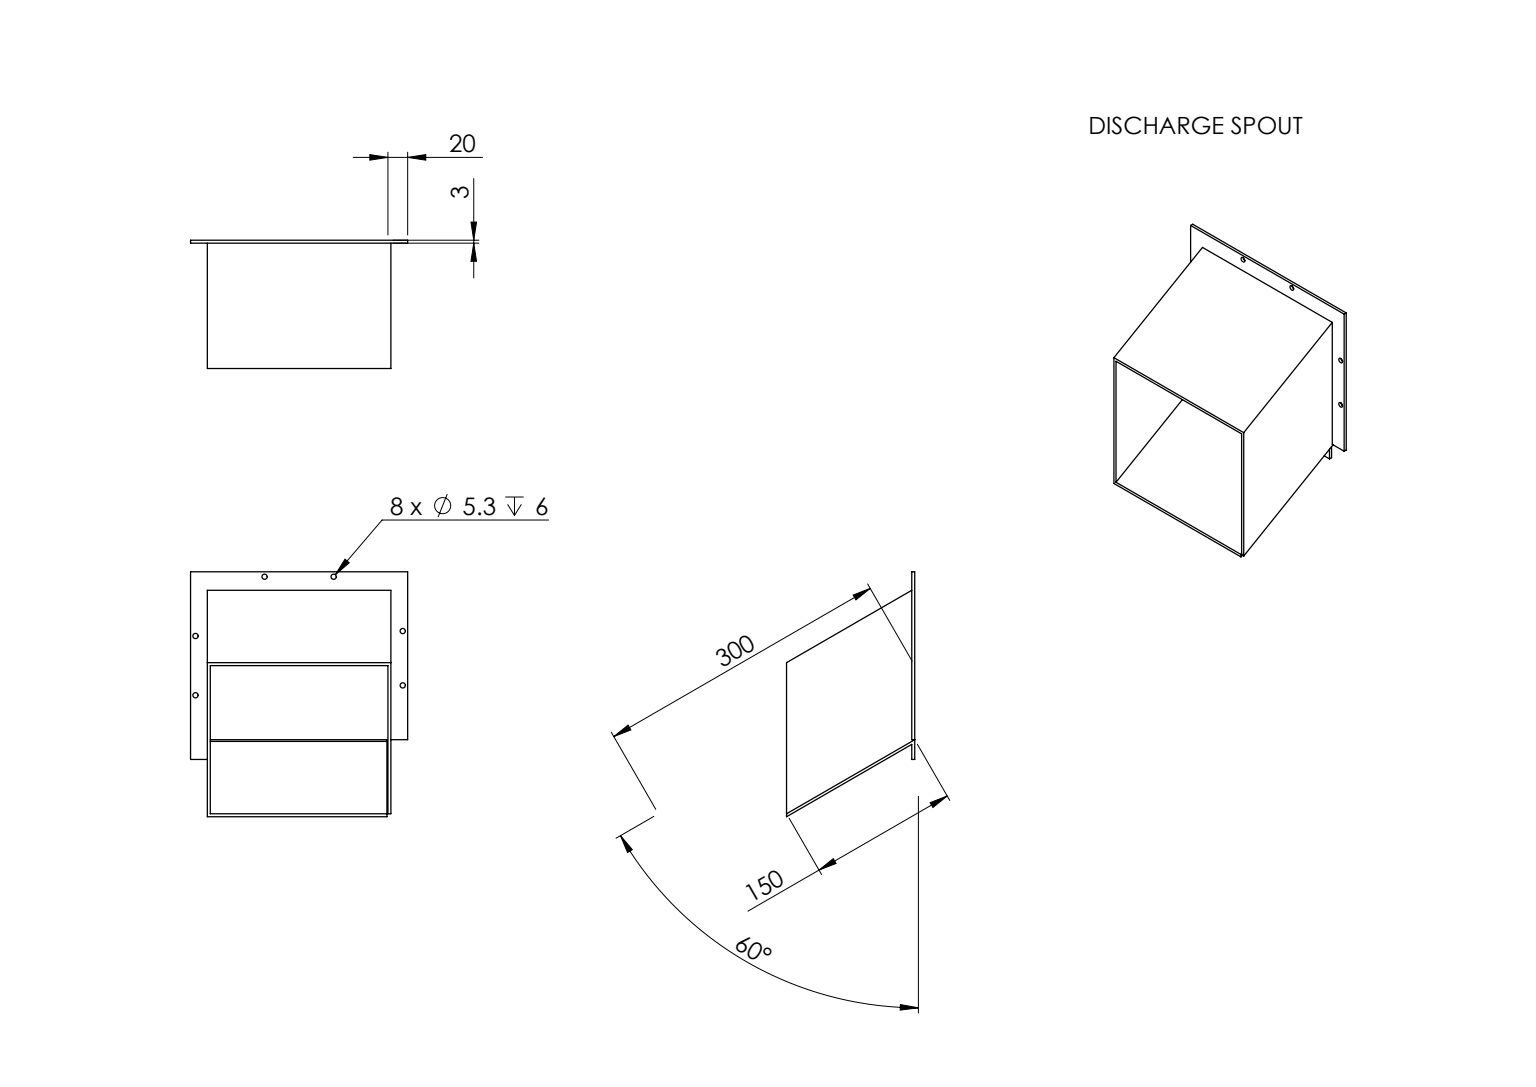
ISO-10303-21;
HEADER;
FILE_DESCRIPTION (('STEP AP214'),
    '1' );
FILE_NAME ('discharge spout.step',
    '2026-10-31T03:46:07',
    ( '' ),
    ( '' ),
    'SwSTEP 2.0',
    'SolidWorks 2026',
    '' );
FILE_SCHEMA (( 'AUTOMOTIVE_DESIGN' ));
ENDSEC;

DATA;
#16=VECTOR ( 'NONE', #9447, 1000.000000000000114 ) ;
#34=EDGE_LOOP ( 'NONE', ( #18835, #10262, #758, #19921 ) ) ;
#69=CARTESIAN_POINT ( 'NONE',  ( 107.6499999999999631, -19.99999999999998934, 0.000000000000000000 ) ) ;
#98=CARTESIAN_POINT ( 'NONE',  ( 110.0000000000000000, 95.00000000000000000, 3.000000000000000000 ) ) ;
#118=ORIENTED_EDGE ( 'NONE', *, *, #9891, .T. ) ;
#138=ADVANCED_FACE ( 'NONE', ( #8828 ), #23557, .F. ) ;
#140=FACE_BOUND ( 'NONE', #2354, .T. ) ;
#151=ORIENTED_EDGE ( 'NONE', *, *, #12197, .F. ) ;
#172=LINE ( 'NONE', #13494, #7239 ) ;
#194=DIRECTION ( 'NONE',  ( -0.000000000000000000, -0.000000000000000000, -1.000000000000000000 ) ) ;
#248=CARTESIAN_POINT ( 'NONE',  ( 37.64999999999997726, 90.00000000000000000, 3.000000000000001332 ) ) ;
#272=AXIS2_PLACEMENT_3D ( 'NONE', #19856, #3615, #4354 ) ;
#301=VERTEX_POINT ( 'NONE', #17262 ) ;
#302=DIRECTION ( 'NONE',  ( 0.000000000000000000, 0.000000000000000000, -1.000000000000000000 ) ) ;
#304=DIRECTION ( 'NONE',  ( -1.000000000000000000, -0.000000000000000000, 0.000000000000000000 ) ) ;
#308=DIRECTION ( 'NONE',  ( 0.000000000000000000, 0.000000000000000000, -1.000000000000000000 ) ) ;
#325=ADVANCED_FACE ( 'NONE', ( #8567 ), #12223, .F. ) ;
#334=LINE ( 'NONE', #15199, #11800 ) ;
#348=FACE_OUTER_BOUND ( 'NONE', #9834, .T. ) ;
#359=VECTOR ( 'NONE', #6487, 1000.000000000000000 ) ;
#406=LINE ( 'NONE', #11777, #11576 ) ;
#442=VERTEX_POINT ( 'NONE', #8210 ) ;
#443=DIRECTION ( 'NONE',  ( -1.000000000000000000, 0.000000000000000000, 0.000000000000000000 ) ) ;
#498=DIRECTION ( 'NONE',  ( -0.000000000000000000, 0.000000000000000000, -1.000000000000000000 ) ) ;
#508=CARTESIAN_POINT ( 'NONE',  ( -90.00000000000000000, -76.73205080756885366, 3.000000000000002665 ) ) ;
#509=ORIENTED_EDGE ( 'NONE', *, *, #16797, .F. ) ;
#528=CARTESIAN_POINT ( 'NONE',  ( -90.00000000000000000, 75.00000000000001421, 0.000000000000000000 ) ) ;
#532=ORIENTED_EDGE ( 'NONE', *, *, #21218, .F. ) ;
#542=CARTESIAN_POINT ( 'NONE',  ( 102.3500000000000227, 35.00000000000000000, 0.000000000000000000 ) ) ;
#557=FACE_OUTER_BOUND ( 'NONE', #1366, .T. ) ;
#565=EDGE_LOOP ( 'NONE', ( #2782, #21644, #4251, #22366 ) ) ;
#571=CIRCLE ( 'NONE', #7503, 2.649999999999971934 ) ;
#587=DIRECTION ( 'NONE',  ( -6.676953772165163028E-17, -0.8660254037844398178, -0.4999999999999980571 ) ) ;
#655=CIRCLE ( 'NONE', #14181, 2.649999999999971934 ) ;
#661=CARTESIAN_POINT ( 'NONE',  ( -90.00000000000000000, -79.73205080756885366, 3.000000000000002665 ) ) ;
#707=ORIENTED_EDGE ( 'NONE', *, *, #13202, .F. ) ;
#714=ORIENTED_EDGE ( 'NONE', *, *, #23299, .F. ) ;
#722=AXIS2_PLACEMENT_3D ( 'NONE', #1603, #20182, #21658 ) ;
#758=ORIENTED_EDGE ( 'NONE', *, *, #16405, .T. ) ;
#773=DIRECTION ( 'NONE',  ( 0.000000000000000000, 0.000000000000000000, -1.000000000000000000 ) ) ;
#783=CARTESIAN_POINT ( 'NONE',  ( 89.00000000000000000, -74.99999999999998579, 3.000000000000000000 ) ) ;
#805=ORIENTED_EDGE ( 'NONE', *, *, #3197, .T. ) ;
#826=ORIENTED_EDGE ( 'NONE', *, *, #2161, .F. ) ;
#836=ORIENTED_EDGE ( 'NONE', *, *, #6196, .T. ) ;
#843=EDGE_CURVE ( 'NONE', #22443, #6335, #8908, .T. ) ;
#878=DIRECTION ( 'NONE',  ( -0.000000000000000000, -0.000000000000000000, 1.000000000000000000 ) ) ;
#901=EDGE_CURVE ( 'NONE', #19530, #15233, #571, .T. ) ;
#935=AXIS2_PLACEMENT_3D ( 'NONE', #10391, #13792, #16052 ) ;
#961=ORIENTED_EDGE ( 'NONE', *, *, #22708, .T. ) ;
#977=AXIS2_PLACEMENT_3D ( 'NONE', #2583, #10105, #18756 ) ;
#994=EDGE_CURVE ( 'NONE', #13225, #7372, #14096, .T. ) ;
#996=LINE ( 'NONE', #12058, #1812 ) ;
#1064=VECTOR ( 'NONE', #2222, 1000.000000000000114 ) ;
#1098=VECTOR ( 'NONE', #7006, 1000.000000000000000 ) ;
#1143=VECTOR ( 'NONE', #17947, 1000.000000000000000 ) ;
#1146=FACE_OUTER_BOUND ( 'NONE', #5619, .T. ) ;
#1171=CARTESIAN_POINT ( 'NONE',  ( 90.00000000000000000, 2.914335439641035919E-13, 129.9038105676659711 ) ) ;
#1217=CARTESIAN_POINT ( 'NONE',  ( 110.0000000000000000, -74.99999999999998579, 0.000000000000000000 ) ) ;
#1219=VERTEX_POINT ( 'NONE', #12614 ) ;
#1241=DIRECTION ( 'NONE',  ( -0.000000000000000000, -0.000000000000000000, -1.000000000000000000 ) ) ;
#1262=CARTESIAN_POINT ( 'NONE',  ( 90.00000000000000000, 2.914335439641035919E-13, 129.9038105676659711 ) ) ;
#1272=DIRECTION ( 'NONE',  ( -0.000000000000000000, 1.000000000000000000, 0.000000000000000000 ) ) ;
#1276=DIRECTION ( 'NONE',  ( 0.000000000000000000, 0.000000000000000000, -1.000000000000000000 ) ) ;
#1286=CARTESIAN_POINT ( 'NONE',  ( 105.0000000000000000, 35.00000000000000000, 0.000000000000000000 ) ) ;
#1327=VECTOR ( 'NONE', #3793, 1000.000000000000114 ) ;
#1340=EDGE_CURVE ( 'NONE', #2213, #6626, #7845, .T. ) ;
#1358=DIRECTION ( 'NONE',  ( -1.000000000000000000, 7.709882115452476934E-17, 0.000000000000000000 ) ) ;
#1364=DIRECTION ( 'NONE',  ( 0.000000000000000000, 0.000000000000000000, -1.000000000000000000 ) ) ;
#1366=EDGE_LOOP ( 'NONE', ( #4331, #2748, #2855, #13215 ) ) ;
#1381=DIRECTION ( 'NONE',  ( -1.000000000000000000, 0.000000000000000000, -0.000000000000000000 ) ) ;
#1397=FACE_OUTER_BOUND ( 'NONE', #1757, .T. ) ;
#1404=FACE_OUTER_BOUND ( 'NONE', #16223, .T. ) ;
#1408=CARTESIAN_POINT ( 'NONE',  ( 24.33333333333333215, -89.99999999999998579, 3.000000000000000000 ) ) ;
#1410=ORIENTED_EDGE ( 'NONE', *, *, #16821, .T. ) ;
#1419=ORIENTED_EDGE ( 'NONE', *, *, #7745, .T. ) ;
#1433=DIRECTION ( 'NONE',  ( -0.000000000000000000, -1.000000000000000000, 0.000000000000000000 ) ) ;
#1442=AXIS2_PLACEMENT_3D ( 'NONE', #13504, #3692, #20685 ) ;
#1476=CIRCLE ( 'NONE', #6881, 2.649999999999985700 ) ;
#1545=AXIS2_PLACEMENT_3D ( 'NONE', #14639, #21749, #20056 ) ;
#1552=DIRECTION ( 'NONE',  ( -0.000000000000000000, -0.000000000000000000, 1.000000000000000000 ) ) ;
#1559=DIRECTION ( 'NONE',  ( 1.000000000000000000, 0.000000000000000000, 0.000000000000000000 ) ) ;
#1568=LINE ( 'NONE', #17988, #14694 ) ;
#1603=CARTESIAN_POINT ( 'NONE',  ( 105.0000000000000000, -19.99999999999998934, 0.000000000000000000 ) ) ;
#1607=EDGE_LOOP ( 'NONE', ( #12718, #7709, #16085, #5672 ) ) ;
#1617=VERTEX_POINT ( 'NONE', #98 ) ;
#1649=EDGE_LOOP ( 'NONE', ( #11565, #23446, #13980, #11039 ) ) ;
#1652=EDGE_CURVE ( 'NONE', #16805, #2178, #14106, .T. ) ;
#1677=CARTESIAN_POINT ( 'NONE',  ( -37.68333333333335844, -89.99999999999997158, 3.000000000000000000 ) ) ;
#1680=CARTESIAN_POINT ( 'NONE',  ( -90.00000000000000000, -94.99999999999998579, 3.000000000000000000 ) ) ;
#1724=EDGE_CURVE ( 'NONE', #16388, #15256, #334, .T. ) ;
#1746=VECTOR ( 'NONE', #9787, 1000.000000000000000 ) ;
#1757=EDGE_LOOP ( 'NONE', ( #8882, #20556, #17821, #15590, #12226, #23679, #18207, #10724, #1419, #19201, #18727 ) ) ;
#1810=ORIENTED_EDGE ( 'NONE', *, *, #19149, .F. ) ;
#1812=VECTOR ( 'NONE', #22970, 1000.000000000000000 ) ;
#1838=CARTESIAN_POINT ( 'NONE',  ( 89.00000000000000000, -149.9999999999996874, 129.9038105676659711 ) ) ;
#1879=PRODUCT_DEFINITION_SHAPE ( 'NONE', 'NONE',  #4601 ) ;
#1922=ORIENTED_EDGE ( 'NONE', *, *, #14781, .F. ) ;
#1929=DIRECTION ( 'NONE',  ( 0.000000000000000000, 0.4999999999999979461, -0.8660254037844397068 ) ) ;
#1955=CARTESIAN_POINT ( 'NONE',  ( -90.00000000000000000, -74.99999999999998579, 0.000000000000000000 ) ) ;
#2036=DIRECTION ( 'NONE',  ( 0.000000000000000000, 1.000000000000000000, 0.000000000000000000 ) ) ;
#2060=ORIENTED_EDGE ( 'NONE', *, *, #9485, .F. ) ;
#2098=CARTESIAN_POINT ( 'NONE',  ( -93.00000000000000000, 3.053113317719180486E-13, 129.9038105676659711 ) ) ;
#2103=LINE ( 'NONE', #22396, #1327 ) ;
#2114=LINE ( 'NONE', #15436, #11916 ) ;
#2130=CARTESIAN_POINT ( 'NONE',  ( -102.3500000000000227, -29.99999999999998579, 3.000000000000000000 ) ) ;
#2140=ORIENTED_EDGE ( 'NONE', *, *, #17933, .F. ) ;
#2161=EDGE_CURVE ( 'NONE', #11272, #13966, #5851, .T. ) ;
#2178=VERTEX_POINT ( 'NONE', #13376 ) ;
#2189=VECTOR ( 'NONE', #10752, 1000.000000000000000 ) ;
#2213=VERTEX_POINT ( 'NONE', #4513 ) ;
#2215=ORIENTED_EDGE ( 'NONE', *, *, #19914, .T. ) ;
#2222=DIRECTION ( 'NONE',  ( -0.000000000000000000, 0.4999999999999979461, -0.8660254037844397068 ) ) ;
#2233=ORIENTED_EDGE ( 'NONE', *, *, #19149, .T. ) ;
#2259=DIRECTION ( 'NONE',  ( -0.000000000000000000, 0.8660254037844398178, 0.4999999999999980571 ) ) ;
#2276=CARTESIAN_POINT ( 'NONE',  ( -90.00000000000000000, 3.053113317719180486E-13, 129.9038105676659711 ) ) ;
#2354=EDGE_LOOP ( 'NONE', ( #7769, #2060 ) ) ;
#2372=EDGE_LOOP ( 'NONE', ( #23298, #19118, #826, #16435 ) ) ;
#2377=CARTESIAN_POINT ( 'NONE',  ( 93.00000000000000000, 3.000000000000280220, 129.9038105676659711 ) ) ;
#2378=ADVANCED_FACE ( 'NONE', ( #9097 ), #5469, .F. ) ;
#2389=EDGE_CURVE ( 'NONE', #2213, #16388, #11171, .T. ) ;
#2413=DIRECTION ( 'NONE',  ( 1.000000000000000000, 0.000000000000000000, -0.000000000000000000 ) ) ;
#2416=EDGE_LOOP ( 'NONE', ( #12908, #4600, #9788, #20832 ) ) ;
#2427=DIRECTION ( 'NONE',  ( -0.000000000000000000, -0.000000000000000000, 1.000000000000000000 ) ) ;
#2435=CIRCLE ( 'NONE', #10954, 2.649999999999971934 ) ;
#2446=EDGE_LOOP ( 'NONE', ( #23698, #9910, #9443, #10299 ) ) ;
#2474=DIRECTION ( 'NONE',  ( 1.000000000000000000, 0.000000000000000000, 0.000000000000000000 ) ) ;
#2477=CARTESIAN_POINT ( 'NONE',  ( 105.0000000000000000, -19.99999999999998934, 3.000000000000001332 ) ) ;
#2487=AXIS2_PLACEMENT_3D ( 'NONE', #16846, #304, #20575 ) ;
#2493=ORIENTED_EDGE ( 'NONE', *, *, #16579, .T. ) ;
#2539=( LENGTH_UNIT ( ) NAMED_UNIT ( * ) SI_UNIT ( .MILLI., .METRE. ) );
#2563=AXIS2_PLACEMENT_3D ( 'NONE', #20779, #22586, #11657 ) ;
#2583=CARTESIAN_POINT ( 'NONE',  ( -105.0000000000000142, 30.00000000000001421, 3.000000000000000000 ) ) ;
#2585=DIRECTION ( 'NONE',  ( -0.000000000000000000, 0.4999999999999979461, -0.8660254037844397068 ) ) ;
#2594=LINE ( 'NONE', #11945, #16704 ) ;
#2624=FACE_OUTER_BOUND ( 'NONE', #20466, .T. ) ;
#2656=FACE_OUTER_BOUND ( 'NONE', #3132, .T. ) ;
#2697=AXIS2_PLACEMENT_3D ( 'NONE', #9721, #15396, #17076 ) ;
#2731=ORIENTED_EDGE ( 'NONE', *, *, #843, .F. ) ;
#2736=VERTEX_POINT ( 'NONE', #8483 ) ;
#2748=ORIENTED_EDGE ( 'NONE', *, *, #13603, .T. ) ;
#2751=DIRECTION ( 'NONE',  ( 0.000000000000000000, 0.000000000000000000, -1.000000000000000000 ) ) ;
#2771=CARTESIAN_POINT ( 'NONE',  ( 93.00000000000000000, -149.9999999999996874, 3.000000000000002665 ) ) ;
#2773=ADVANCED_FACE ( 'NONE', ( #22721 ), #6190, .F. ) ;
#2782=ORIENTED_EDGE ( 'NONE', *, *, #15460, .F. ) ;
#2794=AXIS2_PLACEMENT_3D ( 'NONE', #15332, #2259, #4328 ) ;
#2795=DIRECTION ( 'NONE',  ( -0.000000000000000000, -0.000000000000000000, 1.000000000000000000 ) ) ;
#2819=DIRECTION ( 'NONE',  ( 1.000000000000000000, 0.000000000000000000, 0.000000000000000000 ) ) ;
#2820=CARTESIAN_POINT ( 'NONE',  ( 89.00000000000000000, -149.9999999999996874, 129.9038105676659711 ) ) ;
#2855=ORIENTED_EDGE ( 'NONE', *, *, #20545, .T. ) ;
#2856=AXIS2_PLACEMENT_3D ( 'NONE', #6457, #20954, #11818 ) ;
#2915=DIRECTION ( 'NONE',  ( -0.000000000000000000, -0.000000000000000000, 1.000000000000000000 ) ) ;
#2930=VECTOR ( 'NONE', #10906, 1000.000000000000000 ) ;
#2948=LINE ( 'NONE', #16020, #14312 ) ;
#2954=FACE_BOUND ( 'NONE', #11229, .T. ) ;
#2963=CARTESIAN_POINT ( 'NONE',  ( 34.99999999999999289, 90.00000000000000000, 3.000000000000000000 ) ) ;
#2993=EDGE_LOOP ( 'NONE', ( #20270, #13924, #8741, #2493 ) ) ;
#2996=EDGE_CURVE ( 'NONE', #6747, #442, #7706, .T. ) ;
#3019=CARTESIAN_POINT ( 'NONE',  ( 102.3500000000000227, 35.00000000000000000, 3.000000000000000000 ) ) ;
#3021=ORIENTED_EDGE ( 'NONE', *, *, #9056, .T. ) ;
#3023=PLANE ( 'NONE',  #7333 ) ;
#3026=LINE ( 'NONE', #10557, #14282 ) ;
#3028=EDGE_LOOP ( 'NONE', ( #16211, #16269, #12851, #22501 ) ) ;
#3057=DIRECTION ( 'NONE',  ( -0.000000000000000000, -0.000000000000000000, 1.000000000000000000 ) ) ;
#3058=VERTEX_POINT ( 'NONE', #4789 ) ;
#3086=EDGE_CURVE ( 'NONE', #21146, #19747, #19634, .T. ) ;
#3120=DIRECTION ( 'NONE',  ( -1.000000000000000000, 0.000000000000000000, 0.000000000000000000 ) ) ;
#3132=EDGE_LOOP ( 'NONE', ( #3290, #805, #21657, #11861, #5062, #18814 ) ) ;
#3167=ORIENTED_EDGE ( 'NONE', *, *, #23772, .F. ) ;
#3171=AXIS2_PLACEMENT_3D ( 'NONE', #7719, #587, #18797 ) ;
#3183=ORIENTED_EDGE ( 'NONE', *, *, #14869, .F. ) ;
#3196=ORIENTED_EDGE ( 'NONE', *, *, #18555, .F. ) ;
#3197=EDGE_CURVE ( 'NONE', #15650, #11272, #16145, .T. ) ;
#3204=CARTESIAN_POINT ( 'NONE',  ( 90.00000000000000000, 75.00000000000000000, 0.000000000000000000 ) ) ;
#3206=CARTESIAN_POINT ( 'NONE',  ( 93.00000000000000000, 3.000000000000280220, 129.9038105676659711 ) ) ;
#3245=ADVANCED_FACE ( 'NONE', ( #3451 ), #3322, .F. ) ;
#3246=ORIENTED_EDGE ( 'NONE', *, *, #19914, .F. ) ;
#3248=ADVANCED_FACE ( 'NONE', ( #14461 ), #21800, .F. ) ;
#3284=VERTEX_POINT ( 'NONE', #4868 ) ;
#3290=ORIENTED_EDGE ( 'NONE', *, *, #12244, .T. ) ;
#3319=FACE_BOUND ( 'NONE', #8470, .T. ) ;
#3322=PLANE ( 'NONE',  #18081 ) ;
#3333=ORIENTED_EDGE ( 'NONE', *, *, #19966, .F. ) ;
#3412=EDGE_LOOP ( 'NONE', ( #21473, #3196 ) ) ;
#3451=FACE_OUTER_BOUND ( 'NONE', #5420, .T. ) ;
#3563=CARTESIAN_POINT ( 'NONE',  ( -37.68333333333334423, -89.99999999999997158, 3.000000000000001332 ) ) ;
#3599=LINE ( 'NONE', #6774, #2930 ) ;
#3606=PLANE ( 'NONE',  #8296 ) ;
#3615=DIRECTION ( 'NONE',  ( 0.000000000000000000, 0.000000000000000000, -1.000000000000000000 ) ) ;
#3625=AXIS2_PLACEMENT_3D ( 'NONE', #22941, #2427, #20207 ) ;
#3637=AXIS2_PLACEMENT_3D ( 'NONE', #21825, #10886, #18102 ) ;
#3654=LINE ( 'NONE', #5376, #15818 ) ;
#3666=VERTEX_POINT ( 'NONE', #542 ) ;
#3692=DIRECTION ( 'NONE',  ( -6.676953772165163028E-17, -0.8660254037844398178, -0.4999999999999980016 ) ) ;
#3729=CARTESIAN_POINT ( 'NONE',  ( 34.99999999999999289, 90.00000000000000000, 0.000000000000000000 ) ) ;
#3731=EDGE_CURVE ( 'NONE', #20709, #23021, #16956, .T. ) ;
#3742=FACE_BOUND ( 'NONE', #15940, .T. ) ;
#3769=DIRECTION ( 'NONE',  ( 1.000000000000000000, 0.000000000000000000, 0.000000000000000000 ) ) ;
#3793=DIRECTION ( 'NONE',  ( -0.000000000000000000, 0.4999999999999979461, -0.8660254037844397068 ) ) ;
#3865=DIRECTION ( 'NONE',  ( -1.000000000000000000, 0.000000000000000000, 0.000000000000000000 ) ) ;
#3903=DIRECTION ( 'NONE',  ( -0.000000000000000000, -0.000000000000000000, 1.000000000000000000 ) ) ;
#3916=CARTESIAN_POINT ( 'NONE',  ( 0.000000000000000000, -74.99999999999970157, 129.9038105676659711 ) ) ;
#4023=VECTOR ( 'NONE', #14170, 1000.000000000000000 ) ;
#4030=EDGE_LOOP ( 'NONE', ( #6266, #7502, #10158, #12104 ) ) ;
#4035=EDGE_CURVE ( 'NONE', #2736, #3058, #406, .T. ) ;
#4068=LINE ( 'NONE', #14973, #19207 ) ;
#4069=DIRECTION ( 'NONE',  ( 1.000000000000000000, 0.000000000000000000, 0.000000000000000000 ) ) ;
#4077=ORIENTED_EDGE ( 'NONE', *, *, #10372, .F. ) ;
#4087=ORIENTED_EDGE ( 'NONE', *, *, #16821, .F. ) ;
#4088=ORIENTED_EDGE ( 'NONE', *, *, #11255, .T. ) ;
#4107=EDGE_CURVE ( 'NONE', #3666, #12421, #4492, .T. ) ;
#4128=ORIENTED_EDGE ( 'NONE', *, *, #9418, .T. ) ;
#4160=CARTESIAN_POINT ( 'NONE',  ( 24.33333333333333215, -89.99999999999998579, 0.000000000000000000 ) ) ;
#4171=EDGE_LOOP ( 'NONE', ( #3167, #509 ) ) ;
#4192=( NAMED_UNIT ( * ) SI_UNIT ( $, .STERADIAN. ) SOLID_ANGLE_UNIT ( ) );
#4235=FILL_AREA_STYLE_COLOUR ( '', #11233 ) ;
#4251=ORIENTED_EDGE ( 'NONE', *, *, #17095, .F. ) ;
#4263=LINE ( 'NONE', #20799, #6531 ) ;
#4264=CIRCLE ( 'NONE', #7355, 2.649999999999971934 ) ;
#4279=ORIENTED_EDGE ( 'NONE', *, *, #18990, .T. ) ;
#4316=LINE ( 'NONE', #4433, #20402 ) ;
#4328=DIRECTION ( 'NONE',  ( 0.000000000000000000, -0.4999999999999980016, 0.8660254037844397068 ) ) ;
#4329=ORIENTED_EDGE ( 'NONE', *, *, #18850, .F. ) ;
#4331=ORIENTED_EDGE ( 'NONE', *, *, #23772, .T. ) ;
#4354=DIRECTION ( 'NONE',  ( -1.000000000000000000, 0.000000000000000000, 0.000000000000000000 ) ) ;
#4369=DIRECTION ( 'NONE',  ( -0.000000000000000000, 0.4999999999999979461, -0.8660254037844397068 ) ) ;
#4376=ADVANCED_FACE ( 'NONE', ( #16432 ), #3606, .T. ) ;
#4381=ORIENTED_EDGE ( 'NONE', *, *, #12291, .T. ) ;
#4414=ORIENTED_EDGE ( 'NONE', *, *, #21218, .T. ) ;
#4433=CARTESIAN_POINT ( 'NONE',  ( -90.00000000000000000, -94.99999999999998579, 3.000000000000000000 ) ) ;
#4478=DIRECTION ( 'NONE',  ( 1.000000000000000000, 0.000000000000000000, 0.000000000000000000 ) ) ;
#4492=LINE ( 'NONE', #3019, #4023 ) ;
#4513=CARTESIAN_POINT ( 'NONE',  ( 102.3500000000000227, -19.99999999999998934, 0.000000000000000000 ) ) ;
#4536=LINE ( 'NONE', #22881, #10837 ) ;
#4547=ORIENTED_EDGE ( 'NONE', *, *, #4035, .F. ) ;
#4572=ORIENTED_EDGE ( 'NONE', *, *, #14395, .T. ) ;
#4594=EDGE_CURVE ( 'NONE', #3058, #19747, #6279, .T. ) ;
#4600=ORIENTED_EDGE ( 'NONE', *, *, #9120, .T. ) ;
#4601=PRODUCT_DEFINITION ( 'UNKNOWN', '', #19285, #5664 ) ;
#4602=EDGE_CURVE ( 'NONE', #1617, #301, #11872, .T. ) ;
#4621=CARTESIAN_POINT ( 'NONE',  ( 89.00000000000000000, -74.99999999999998579, 3.000000000000000000 ) ) ;
#4661=DIRECTION ( 'NONE',  ( 1.000000000000000000, 0.000000000000000000, 0.000000000000000000 ) ) ;
#4704=DIRECTION ( 'NONE',  ( 0.000000000000000000, 1.000000000000000000, 0.000000000000000000 ) ) ;
#4707=VERTEX_POINT ( 'NONE', #21722 ) ;
#4731=ADVANCED_FACE ( 'NONE', ( #23541 ), #18105, .F. ) ;
#4739=ORIENTED_EDGE ( 'NONE', *, *, #11255, .F. ) ;
#4751=ORIENTED_EDGE ( 'NONE', *, *, #16662, .F. ) ;
#4776=ORIENTED_EDGE ( 'NONE', *, *, #2389, .F. ) ;
#4779=DIRECTION ( 'NONE',  ( 1.000000000000000000, 0.000000000000000000, 0.000000000000000000 ) ) ;
#4789=CARTESIAN_POINT ( 'NONE',  ( 90.00000000000000000, -74.99999999999998579, 0.000000000000000000 ) ) ;
#4839=VERTEX_POINT ( 'NONE', #17450 ) ;
#4848=ADVANCED_FACE ( 'NONE', ( #15175 ), #15296, .F. ) ;
#4868=CARTESIAN_POINT ( 'NONE',  ( 93.00000000000000000, -74.99999999999998579, 0.000000000000000000 ) ) ;
#4954=AXIS2_PLACEMENT_3D ( 'NONE', #5211, #16326, #10916 ) ;
#4983=ORIENTED_EDGE ( 'NONE', *, *, #22838, .F. ) ;
#5021=CARTESIAN_POINT ( 'NONE',  ( 32.35000000000000142, 90.00000000000000000, 3.000000000000001332 ) ) ;
#5030=DIRECTION ( 'NONE',  ( 0.000000000000000000, 1.000000000000000000, 0.000000000000000000 ) ) ;
#5059=ORIENTED_EDGE ( 'NONE', *, *, #9120, .F. ) ;
#5062=ORIENTED_EDGE ( 'NONE', *, *, #17138, .F. ) ;
#5073=VERTEX_POINT ( 'NONE', #2820 ) ;
#5164=ORIENTED_EDGE ( 'NONE', *, *, #3086, .F. ) ;
#5203=ADVANCED_FACE ( 'NONE', ( #17063 ), #9947, .F. ) ;
#5211=CARTESIAN_POINT ( 'NONE',  ( -105.0000000000000000, -29.99999999999998579, 3.000000000000001332 ) ) ;
#5247=VECTOR ( 'NONE', #22265, 1000.000000000000000 ) ;
#5266=CARTESIAN_POINT ( 'NONE',  ( 0.000000000000000000, 0.000000000000000000, 3.000000000000000000 ) ) ;
#5290=ADVANCED_FACE ( 'NONE', ( #11780 ), #19093, .T. ) ;
#5332=LINE ( 'NONE', #8967, #13118 ) ;
#5341=ORIENTED_EDGE ( 'NONE', *, *, #16797, .T. ) ;
#5344=AXIS2_PLACEMENT_3D ( 'NONE', #19132, #22771, #11702 ) ;
#5374=CARTESIAN_POINT ( 'NONE',  ( 107.6499999999999631, 35.00000000000000000, 0.000000000000000000 ) ) ;
#5376=CARTESIAN_POINT ( 'NONE',  ( 110.0000000000000000, -74.99999999999998579, 0.000000000000000000 ) ) ;
#5377=DIRECTION ( 'NONE',  ( -0.000000000000000000, 1.000000000000000000, 0.000000000000000000 ) ) ;
#5417=FACE_OUTER_BOUND ( 'NONE', #23397, .T. ) ;
#5420=EDGE_LOOP ( 'NONE', ( #118, #23693, #15514, #9819, #2731 ) ) ;
#5435=ADVANCED_FACE ( 'NONE', ( #13959 ), #3023, .F. ) ;
#5469=CYLINDRICAL_SURFACE ( 'NONE', #21551, 2.649999999999971934 ) ;
#5500=EDGE_LOOP ( 'NONE', ( #707, #10192 ) ) ;
#5513=VERTEX_POINT ( 'NONE', #11148 ) ;
#5581=EDGE_LOOP ( 'NONE', ( #21984, #3246 ) ) ;
#5593=ADVANCED_FACE ( 'NONE', ( #14409 ), #21853, .F. ) ;
#5607=DIRECTION ( 'NONE',  ( 0.000000000000000000, 0.000000000000000000, -1.000000000000000000 ) ) ;
#5619=EDGE_LOOP ( 'NONE', ( #4983, #9747, #9965, #961 ) ) ;
#5629=DIRECTION ( 'NONE',  ( -1.000000000000000000, 7.709882115452476934E-17, 0.000000000000000000 ) ) ;
#5636=LINE ( 'NONE', #14376, #15059 ) ;
#5655=CIRCLE ( 'NONE', #13018, 2.649999999999971934 ) ;
#5664=PRODUCT_DEFINITION_CONTEXT ( 'detailed design', #7209, 'design' ) ;
#5672=ORIENTED_EDGE ( 'NONE', *, *, #15086, .T. ) ;
#5676=DIRECTION ( 'NONE',  ( -1.000000000000000000, 0.000000000000000000, 0.000000000000000000 ) ) ;
#5682=CARTESIAN_POINT ( 'NONE',  ( -93.00000000000000000, 3.000000000000308198, 129.9038105676659711 ) ) ;
#5704=EDGE_LOOP ( 'NONE', ( #7763, #9804, #14728, #19769 ) ) ;
#5719=CARTESIAN_POINT ( 'NONE',  ( 26.98333333333330231, -89.99999999999998579, 3.000000000000000000 ) ) ;
#5745=ORIENTED_EDGE ( 'NONE', *, *, #20222, .F. ) ;
#5821=DIRECTION ( 'NONE',  ( 0.000000000000000000, 0.000000000000000000, -1.000000000000000000 ) ) ;
#5849=EDGE_CURVE ( 'NONE', #6867, #15717, #14279, .T. ) ;
#5851=LINE ( 'NONE', #9486, #18664 ) ;
#5869=CARTESIAN_POINT ( 'NONE',  ( -110.0000000000000000, 75.00000000000001421, 0.000000000000000000 ) ) ;
#5919=CARTESIAN_POINT ( 'NONE',  ( -110.0000000000000000, 75.00000000000001421, 3.000000000000000000 ) ) ;
#5927=SURFACE_STYLE_USAGE ( .BOTH. , #9558 ) ;
#5930=EDGE_CURVE ( 'NONE', #301, #10091, #1568, .T. ) ;
#5976=EDGE_LOOP ( 'NONE', ( #2140, #15894 ) ) ;
#6030=FACE_OUTER_BOUND ( 'NONE', #2993, .T. ) ;
#6056=EDGE_LOOP ( 'NONE', ( #1810, #7210 ) ) ;
#6063=CARTESIAN_POINT ( 'NONE',  ( 90.00000000000000000, -149.9999999999996874, 129.9038105676659711 ) ) ;
#6067=DIRECTION ( 'NONE',  ( 0.000000000000000000, -1.000000000000000000, 0.000000000000000000 ) ) ;
#6068=CARTESIAN_POINT ( 'NONE',  ( -40.33333333333332860, -89.99999999999997158, 3.000000000000001332 ) ) ;
#6073=VERTEX_POINT ( 'NONE', #11477 ) ;
#6121=VERTEX_POINT ( 'NONE', #12098 ) ;
#6131=VECTOR ( 'NONE', #23378, 1000.000000000000114 ) ;
#6143=AXIS2_PLACEMENT_3D ( 'NONE', #17929, #17680, #4661 ) ;
#6153=CARTESIAN_POINT ( 'NONE',  ( 102.3500000000000227, -19.99999999999998934, 3.000000000000000000 ) ) ;
#6159=CARTESIAN_POINT ( 'NONE',  ( -90.00000000000000000, 3.053113317719180486E-13, 129.9038105676659711 ) ) ;
#6190=CYLINDRICAL_SURFACE ( 'NONE', #14662, 2.649999999999971934 ) ;
#6196=EDGE_CURVE ( 'NONE', #15218, #3666, #4264, .T. ) ;
#6223=FACE_OUTER_BOUND ( 'NONE', #2446, .T. ) ;
#6243=EDGE_LOOP ( 'NONE', ( #15872, #22651, #4128, #4279 ) ) ;
#6263=DIRECTION ( 'NONE',  ( -0.000000000000000000, -0.000000000000000000, 1.000000000000000000 ) ) ;
#6266=ORIENTED_EDGE ( 'NONE', *, *, #8229, .T. ) ;
#6279=LINE ( 'NONE', #14148, #14868 ) ;
#6289=VECTOR ( 'NONE', #12571, 1000.000000000000000 ) ;
#6291=CARTESIAN_POINT ( 'NONE',  ( 93.00000000000000000, -74.99999999999998579, 3.000000000000002665 ) ) ;
#6335=VERTEX_POINT ( 'NONE', #3206 ) ;
#6339=LINE ( 'NONE', #11939, #1064 ) ;
#6344=FACE_BOUND ( 'NONE', #3412, .T. ) ;
#6353=VECTOR ( 'NONE', #17209, 1000.000000000000000 ) ;
#6457=CARTESIAN_POINT ( 'NONE',  ( 24.33333333333333215, -89.99999999999998579, 3.000000000000001332 ) ) ;
#6461=DIRECTION ( 'NONE',  ( 1.000000000000000000, 0.000000000000000000, 0.000000000000000000 ) ) ;
#6484=AXIS2_PLACEMENT_3D ( 'NONE', #11956, #13999, #4779 ) ;
#6487=DIRECTION ( 'NONE',  ( -0.000000000000000000, -0.000000000000000000, -1.000000000000000000 ) ) ;
#6521=DIRECTION ( 'NONE',  ( -0.000000000000000000, -0.000000000000000000, 1.000000000000000000 ) ) ;
#6523=VECTOR ( 'NONE', #21222, 1000.000000000000114 ) ;
#6531=VECTOR ( 'NONE', #6067, 1000.000000000000000 ) ;
#6568=CARTESIAN_POINT ( 'NONE',  ( 105.0000000000000000, -19.99999999999998934, 3.000000000000000000 ) ) ;
#6602=FACE_OUTER_BOUND ( 'NONE', #18038, .T. ) ;
#6626=VERTEX_POINT ( 'NONE', #17349 ) ;
#6638=EDGE_CURVE ( 'NONE', #20854, #13225, #3026, .T. ) ;
#6652=ORIENTED_EDGE ( 'NONE', *, *, #22567, .T. ) ;
#6688=DIRECTION ( 'NONE',  ( -1.000000000000000000, 0.000000000000000000, 0.000000000000000000 ) ) ;
#6696=CARTESIAN_POINT ( 'NONE',  ( 102.3500000000000085, 35.00000000000000000, 3.000000000000001332 ) ) ;
#6709=DIRECTION ( 'NONE',  ( -0.000000000000000000, -0.000000000000000000, -1.000000000000000000 ) ) ;
#6717=VECTOR ( 'NONE', #12099, 1000.000000000000000 ) ;
#6721=FACE_BOUND ( 'NONE', #6056, .T. ) ;
#6747=VERTEX_POINT ( 'NONE', #7248 ) ;
#6774=CARTESIAN_POINT ( 'NONE',  ( 90.00000000000000000, 3.000000000000293987, 129.9038105676659711 ) ) ;
#6867=VERTEX_POINT ( 'NONE', #20523 ) ;
#6881=AXIS2_PLACEMENT_3D ( 'NONE', #6068, #7637, #11669 ) ;
#6899=VECTOR ( 'NONE', #18977, 1000.000000000000000 ) ;
#6928=DIRECTION ( 'NONE',  ( 1.000000000000000000, 0.000000000000000000, 0.000000000000000000 ) ) ;
#6930=EDGE_LOOP ( 'NONE', ( #8491, #13746, #532, #3183, #20332, #1922, #8276, #21726, #7195, #19956 ) ) ;
#7006=DIRECTION ( 'NONE',  ( -0.000000000000000000, -0.000000000000000000, 1.000000000000000000 ) ) ;
#7015=DIRECTION ( 'NONE',  ( 0.000000000000000000, -0.000000000000000000, 1.000000000000000000 ) ) ;
#7076=ORIENTED_EDGE ( 'NONE', *, *, #19966, .T. ) ;
#7195=ORIENTED_EDGE ( 'NONE', *, *, #17095, .T. ) ;
#7209=APPLICATION_CONTEXT ( 'automotive_design' ) ;
#7210=ORIENTED_EDGE ( 'NONE', *, *, #18932, .F. ) ;
#7229=AXIS2_PLACEMENT_3D ( 'NONE', #22057, #773, #9155 ) ;
#7239=VECTOR ( 'NONE', #3903, 1000.000000000000000 ) ;
#7248=CARTESIAN_POINT ( 'NONE',  ( -102.3500000000000227, -29.99999999999998579, 0.000000000000000000 ) ) ;
#7260=ADVANCED_FACE ( 'NONE', ( #10536 ), #19314, .F. ) ;
#7277=VERTEX_POINT ( 'NONE', #12370 ) ;
#7333=AXIS2_PLACEMENT_3D ( 'NONE', #21639, #19694, #18010 ) ;
#7342=ORIENTED_EDGE ( 'NONE', *, *, #6638, .F. ) ;
#7355=AXIS2_PLACEMENT_3D ( 'NONE', #1286, #2751, #17481 ) ;
#7372=VERTEX_POINT ( 'NONE', #16658 ) ;
#7384=PLANE ( 'NONE',  #12520 ) ;
#7391=ORIENTED_EDGE ( 'NONE', *, *, #1724, .T. ) ;
#7453=ORIENTED_EDGE ( 'NONE', *, *, #22252, .F. ) ;
#7473=ADVANCED_FACE ( 'NONE', ( #348 ), #17254, .T. ) ;
#7482=ADVANCED_FACE ( 'NONE', ( #19163 ), #7830, .F. ) ;
#7493=FACE_OUTER_BOUND ( 'NONE', #21611, .T. ) ;
#7497=AXIS2_PLACEMENT_3D ( 'NONE', #12853, #3057, #22082 ) ;
#7502=ORIENTED_EDGE ( 'NONE', *, *, #17738, .T. ) ;
#7503=AXIS2_PLACEMENT_3D ( 'NONE', #17173, #5607, #20785 ) ;
#7504=CARTESIAN_POINT ( 'NONE',  ( -105.0000000000000000, -29.99999999999998579, 0.000000000000000000 ) ) ;
#7517=LINE ( 'NONE', #18166, #16518 ) ;
#7518=ADVANCED_FACE ( 'NONE', ( #18928 ), #22798, .F. ) ;
#7522=ADVANCED_FACE ( 'NONE', ( #2624 ), #22545, .T. ) ;
#7555=CARTESIAN_POINT ( 'NONE',  ( -107.6499999999999915, 30.00000000000001421, 3.000000000000001332 ) ) ;
#7556=AXIS2_PLACEMENT_3D ( 'NONE', #6063, #9826, #17305 ) ;
#7561=ORIENTED_EDGE ( 'NONE', *, *, #13717, .F. ) ;
#7581=CARTESIAN_POINT ( 'NONE',  ( 21.68333333333335844, -89.99999999999998579, 0.000000000000000000 ) ) ;
#7595=AXIS2_PLACEMENT_3D ( 'NONE', #23278, #1552, #21713 ) ;
#7623=EDGE_CURVE ( 'NONE', #3666, #15218, #2435, .T. ) ;
#7637=DIRECTION ( 'NONE',  ( -0.000000000000000000, -0.000000000000000000, 1.000000000000000000 ) ) ;
#7662=AXIS2_PLACEMENT_3D ( 'NONE', #4160, #308, #443 ) ;
#7706=LINE ( 'NONE', #2130, #9298 ) ;
#7707=EDGE_CURVE ( 'NONE', #3284, #15717, #21811, .T. ) ;
#7709=ORIENTED_EDGE ( 'NONE', *, *, #23183, .F. ) ;
#7719=CARTESIAN_POINT ( 'NONE',  ( 90.00000000000000000, 2.914335439641035919E-13, 129.9038105676659711 ) ) ;
#7726=AXIS2_PLACEMENT_3D ( 'NONE', #5266, #8738, #19456 ) ;
#7745=EDGE_CURVE ( 'NONE', #19747, #13550, #9026, .T. ) ;
#7763=ORIENTED_EDGE ( 'NONE', *, *, #12402, .F. ) ;
#7769=ORIENTED_EDGE ( 'NONE', *, *, #18990, .F. ) ;
#7794=CARTESIAN_POINT ( 'NONE',  ( 32.35000000000001563, 90.00000000000000000, 3.000000000000000000 ) ) ;
#7830=CYLINDRICAL_SURFACE ( 'NONE', #15556, 2.649999999999971934 ) ;
#7845=LINE ( 'NONE', #6153, #1746 ) ;
#7862=FILL_AREA_STYLE ('',( #4235 ) ) ;
#7876=VERTEX_POINT ( 'NONE', #7555 ) ;
#7911=EDGE_LOOP ( 'NONE', ( #11886, #14459 ) ) ;
#7946=( LENGTH_UNIT ( ) NAMED_UNIT ( * ) SI_UNIT ( .MILLI., .METRE. ) );
#7978=EDGE_CURVE ( 'NONE', #5513, #8336, #2594, .T. ) ;
#7991=DIRECTION ( 'NONE',  ( 0.000000000000000000, 0.000000000000000000, -1.000000000000000000 ) ) ;
#8056=EDGE_LOOP ( 'NONE', ( #3333, #20649, #9145, #22896 ) ) ;
#8080=DIRECTION ( 'NONE',  ( -0.000000000000000000, -0.000000000000000000, 1.000000000000000000 ) ) ;
#8081=ADVANCED_FACE ( 'NONE', ( #6344, #16796, #140, #11036, #12432, #14214, #3742, #14342, #7493 ), #7384, .F. ) ;
#8084=CIRCLE ( 'NONE', #7662, 2.649999999999971934 ) ;
#8186=ADVANCED_BREP_SHAPE_REPRESENTATION ( '', ( #11885, #11210 ), #22754 ) ;
#8201=LINE ( 'NONE', #10139, #359 ) ;
#8210=CARTESIAN_POINT ( 'NONE',  ( -102.3500000000000085, -29.99999999999998579, 3.000000000000001332 ) ) ;
#8222=FACE_OUTER_BOUND ( 'NONE', #18774, .T. ) ;
#8229=EDGE_CURVE ( 'NONE', #20414, #20433, #13812, .T. ) ;
#8243=DIRECTION ( 'NONE',  ( -0.000000000000000000, 0.000000000000000000, -1.000000000000000000 ) ) ;
#8276=ORIENTED_EDGE ( 'NONE', *, *, #19191, .F. ) ;
#8285=EDGE_CURVE ( 'NONE', #442, #14560, #9928, .T. ) ;
#8296=AXIS2_PLACEMENT_3D ( 'NONE', #18007, #14407, #1929 ) ;
#8336=VERTEX_POINT ( 'NONE', #12016 ) ;
#8339=SHAPE_REPRESENTATION_RELATIONSHIP ( 'NONE' , 'NONE' ,  #21947, #8186 ) ;
#8344=ORIENTED_EDGE ( 'NONE', *, *, #16367, .T. ) ;
#8345=VECTOR ( 'NONE', #1241, 1000.000000000000000 ) ;
#8369=LINE ( 'NONE', #21399, #8516 ) ;
#8401=ORIENTED_EDGE ( 'NONE', *, *, #9042, .T. ) ;
#8417=CIRCLE ( 'NONE', #4954, 2.649999999999985700 ) ;
#8434=EDGE_LOOP ( 'NONE', ( #21020, #19042 ) ) ;
#8436=CARTESIAN_POINT ( 'NONE',  ( 89.00000000000000000, -152.9999999999996874, 129.9038105676659711 ) ) ;
#8450=ORIENTED_EDGE ( 'NONE', *, *, #1340, .F. ) ;
#8467=( NAMED_UNIT ( * ) PLANE_ANGLE_UNIT ( ) SI_UNIT ( $, .RADIAN. ) );
#8470=EDGE_LOOP ( 'NONE', ( #21110, #14880 ) ) ;
#8483=CARTESIAN_POINT ( 'NONE',  ( 90.00000000000000000, -149.9999999999996874, 129.9038105676659711 ) ) ;
#8485=EDGE_CURVE ( 'NONE', #15233, #23406, #23657, .T. ) ;
#8491=ORIENTED_EDGE ( 'NONE', *, *, #12765, .T. ) ;
#8516=VECTOR ( 'NONE', #21049, 1000.000000000000000 ) ;
#8525=CYLINDRICAL_SURFACE ( 'NONE', #21758, 2.649999999999971934 ) ;
#8545=DIRECTION ( 'NONE',  ( -0.000000000000000000, -0.000000000000000000, -1.000000000000000000 ) ) ;
#8567=FACE_OUTER_BOUND ( 'NONE', #18944, .T. ) ;
#8662=CYLINDRICAL_SURFACE ( 'NONE', #9966, 2.649999999999971934 ) ;
#8684=CARTESIAN_POINT ( 'NONE',  ( -32.35000000000004405, 90.00000000000001421, 3.000000000000000000 ) ) ;
#8738=DIRECTION ( 'NONE',  ( 0.000000000000000000, 0.000000000000000000, -1.000000000000000000 ) ) ;
#8741=ORIENTED_EDGE ( 'NONE', *, *, #2161, .T. ) ;
#8769=VECTOR ( 'NONE', #22313, 1000.000000000000000 ) ;
#8777=ORIENTED_EDGE ( 'NONE', *, *, #15086, .F. ) ;
#8803=AXIS2_PLACEMENT_3D ( 'NONE', #12895, #16128, #20202 ) ;
#8828=FACE_OUTER_BOUND ( 'NONE', #1607, .T. ) ;
#8848=DIRECTION ( 'NONE',  ( -0.000000000000000000, -0.000000000000000000, 1.000000000000000000 ) ) ;
#8882=ORIENTED_EDGE ( 'NONE', *, *, #20222, .T. ) ;
#8906=MECHANICAL_DESIGN_GEOMETRIC_PRESENTATION_REPRESENTATION('',(#13111),#16932);
#8908=LINE ( 'NONE', #10601, #16769 ) ;
#8913=FACE_BOUND ( 'NONE', #4171, .T. ) ;
#8916=CARTESIAN_POINT ( 'NONE',  ( 93.00000000000000000, -149.9999999999996874, 129.9038105676659711 ) ) ;
#8920=DIRECTION ( 'NONE',  ( 1.000000000000000000, 0.000000000000000000, 0.000000000000000000 ) ) ;
#8967=CARTESIAN_POINT ( 'NONE',  ( 110.0000000000000000, -74.99999999999998579, 3.000000000000000000 ) ) ;
#8969=LINE ( 'NONE', #14310, #21935 ) ;
#8998=ORIENTED_EDGE ( 'NONE', *, *, #22708, .F. ) ;
#9026=LINE ( 'NONE', #18197, #17480 ) ;
#9042=EDGE_CURVE ( 'NONE', #21146, #11458, #2114, .T. ) ;
#9056=EDGE_CURVE ( 'NONE', #9146, #5513, #19137, .T. ) ;
#9097=FACE_OUTER_BOUND ( 'NONE', #15275, .T. ) ;
#9120=EDGE_CURVE ( 'NONE', #23021, #16805, #19736, .T. ) ;
#9145=ORIENTED_EDGE ( 'NONE', *, *, #10817, .T. ) ;
#9146=VERTEX_POINT ( 'NONE', #14218 ) ;
#9153=ORIENTED_EDGE ( 'NONE', *, *, #8285, .T. ) ;
#9155=DIRECTION ( 'NONE',  ( -1.000000000000000000, 0.000000000000000000, 0.000000000000000000 ) ) ;
#9182=VECTOR ( 'NONE', #16251, 1000.000000000000000 ) ;
#9229=ORIENTED_EDGE ( 'NONE', *, *, #22436, .T. ) ;
#9239=FACE_OUTER_BOUND ( 'NONE', #19216, .T. ) ;
#9270=CARTESIAN_POINT ( 'NONE',  ( -37.64999999999999147, 90.00000000000001421, 0.000000000000000000 ) ) ;
#9288=ORIENTED_EDGE ( 'NONE', *, *, #15677, .T. ) ;
#9298=VECTOR ( 'NONE', #9522, 1000.000000000000000 ) ;
#9316=EDGE_CURVE ( 'NONE', #16388, #2213, #18404, .T. ) ;
#9338=LINE ( 'NONE', #11290, #16 ) ;
#9361=DIRECTION ( 'NONE',  ( -0.000000000000000000, -0.000000000000000000, 1.000000000000000000 ) ) ;
#9389=CARTESIAN_POINT ( 'NONE',  ( -90.00000000000000000, 3.053113317719180486E-13, 129.9038105676659711 ) ) ;
#9418=EDGE_CURVE ( 'NONE', #20414, #17401, #172, .T. ) ;
#9436=EDGE_CURVE ( 'NONE', #20709, #2178, #13367, .T. ) ;
#9443=ORIENTED_EDGE ( 'NONE', *, *, #21594, .F. ) ;
#9447=DIRECTION ( 'NONE',  ( -0.000000000000000000, 0.4999999999999979461, -0.8660254037844397068 ) ) ;
#9473=CARTESIAN_POINT ( 'NONE',  ( 0.000000000000000000, 0.000000000000000000, 0.000000000000000000 ) ) ;
#9485=EDGE_CURVE ( 'NONE', #7876, #17401, #14676, .T. ) ;
#9486=CARTESIAN_POINT ( 'NONE',  ( -90.00000000000000000, -74.99999999999998579, 3.000000000000000000 ) ) ;
#9497=DIRECTION ( 'NONE',  ( -1.000000000000000000, 0.000000000000000000, -0.000000000000000000 ) ) ;
#9522=DIRECTION ( 'NONE',  ( -0.000000000000000000, -0.000000000000000000, 1.000000000000000000 ) ) ;
#9527=CIRCLE ( 'NONE', #2563, 2.649999999999971934 ) ;
#9544=ORIENTED_EDGE ( 'NONE', *, *, #14781, .T. ) ;
#9558=SURFACE_SIDE_STYLE ('',( #9807 ) ) ;
#9581=DIRECTION ( 'NONE',  ( 1.000000000000000000, 0.000000000000000000, -0.000000000000000000 ) ) ;
#9618=DIRECTION ( 'NONE',  ( 1.000000000000000000, 0.000000000000000000, 0.000000000000000000 ) ) ;
#9621=DIRECTION ( 'NONE',  ( -0.000000000000000000, -0.000000000000000000, 1.000000000000000000 ) ) ;
#9646=AXIS2_PLACEMENT_3D ( 'NONE', #15888, #1364, #6688 ) ;
#9693=ORIENTED_EDGE ( 'NONE', *, *, #11074, .T. ) ;
#9696=( NAMED_UNIT ( * ) SI_UNIT ( $, .STERADIAN. ) SOLID_ANGLE_UNIT ( ) );
#9701=CARTESIAN_POINT ( 'NONE',  ( 21.68333333333334423, -89.99999999999998579, 3.000000000000001332 ) ) ;
#9717=ORIENTED_EDGE ( 'NONE', *, *, #4594, .F. ) ;
#9721=CARTESIAN_POINT ( 'NONE',  ( -105.0000000000000142, 30.00000000000001421, 3.000000000000001332 ) ) ;
#9740=CARTESIAN_POINT ( 'NONE',  ( 34.99999999999999289, 90.00000000000000000, 3.000000000000000000 ) ) ;
#9747=ORIENTED_EDGE ( 'NONE', *, *, #901, .T. ) ;
#9787=DIRECTION ( 'NONE',  ( -0.000000000000000000, -0.000000000000000000, 1.000000000000000000 ) ) ;
#9788=ORIENTED_EDGE ( 'NONE', *, *, #1652, .T. ) ;
#9804=ORIENTED_EDGE ( 'NONE', *, *, #9891, .F. ) ;
#9807=SURFACE_STYLE_FILL_AREA ( #7862 ) ;
#9819=ORIENTED_EDGE ( 'NONE', *, *, #14261, .F. ) ;
#9826=DIRECTION ( 'NONE',  ( -1.000000000000000000, 0.000000000000000000, 0.000000000000000000 ) ) ;
#9834=EDGE_LOOP ( 'NONE', ( #17408, #9229, #10762, #4414 ) ) ;
#9862=CARTESIAN_POINT ( 'NONE',  ( 34.99999999999999289, 90.00000000000000000, 3.000000000000001332 ) ) ;
#9880=VECTOR ( 'NONE', #15295, 1000.000000000000000 ) ;
#9891=EDGE_CURVE ( 'NONE', #22443, #3284, #9338, .T. ) ;
#9893=CARTESIAN_POINT ( 'NONE',  ( -42.98333333333330586, -89.99999999999997158, 0.000000000000000000 ) ) ;
#9910=ORIENTED_EDGE ( 'NONE', *, *, #15527, .F. ) ;
#9928=CIRCLE ( 'NONE', #17610, 2.649999999999985700 ) ;
#9946=UNCERTAINTY_MEASURE_WITH_UNIT (LENGTH_MEASURE( 1.000000000000000082E-05 ), #2539, 'distance_accuracy_value', 'NONE');
#9947=PLANE ( 'NONE',  #17203 ) ;
#9965=ORIENTED_EDGE ( 'NONE', *, *, #8485, .T. ) ;
#9966=AXIS2_PLACEMENT_3D ( 'NONE', #2963, #19639, #8920 ) ;
#9974=LINE ( 'NONE', #783, #6353 ) ;
#9975=ORIENTED_EDGE ( 'NONE', *, *, #17385, .T. ) ;
#9980=VERTEX_POINT ( 'NONE', #8436 ) ;
#9996=ORIENTED_EDGE ( 'NONE', *, *, #15677, .F. ) ;
#10009=LINE ( 'NONE', #2377, #6523 ) ;
#10020=CARTESIAN_POINT ( 'NONE',  ( 105.0000000000000000, 35.00000000000000000, 0.000000000000000000 ) ) ;
#10032=AXIS2_PLACEMENT_3D ( 'NONE', #5919, #2413, #498 ) ;
#10056=PLANE ( 'NONE',  #10032 ) ;
#10091=VERTEX_POINT ( 'NONE', #11342 ) ;
#10095=CARTESIAN_POINT ( 'NONE',  ( 89.00000000000000000, -94.99999999999998579, 3.000000000000000000 ) ) ;
#10105=DIRECTION ( 'NONE',  ( -0.000000000000000000, -0.000000000000000000, 1.000000000000000000 ) ) ;
#10139=CARTESIAN_POINT ( 'NONE',  ( 89.00000000000000000, -94.99999999999998579, 3.000000000000000000 ) ) ;
#10148=LINE ( 'NONE', #8684, #2189 ) ;
#10158=ORIENTED_EDGE ( 'NONE', *, *, #9485, .T. ) ;
#10184=CARTESIAN_POINT ( 'NONE',  ( -102.3500000000000369, 30.00000000000001421, 0.000000000000000000 ) ) ;
#10192=ORIENTED_EDGE ( 'NONE', *, *, #1652, .F. ) ;
#10245=VECTOR ( 'NONE', #8545, 1000.000000000000000 ) ;
#10254=CARTESIAN_POINT ( 'NONE',  ( 105.0000000000000000, 35.00000000000000000, 3.000000000000001332 ) ) ;
#10262=ORIENTED_EDGE ( 'NONE', *, *, #22838, .T. ) ;
#10277=ORIENTED_EDGE ( 'NONE', *, *, #4107, .T. ) ;
#10299=ORIENTED_EDGE ( 'NONE', *, *, #13717, .T. ) ;
#10314=DIRECTION ( 'NONE',  ( 1.000000000000000000, 0.000000000000000000, 0.000000000000000000 ) ) ;
#10341=VECTOR ( 'NONE', #10345, 1000.000000000000000 ) ;
#10345=DIRECTION ( 'NONE',  ( -0.000000000000000000, -0.000000000000000000, 1.000000000000000000 ) ) ;
#10372=EDGE_CURVE ( 'NONE', #16588, #1219, #2948, .T. ) ;
#10384=EDGE_LOOP ( 'NONE', ( #8450, #23425, #7391, #18815 ) ) ;
#10391=CARTESIAN_POINT ( 'NONE',  ( 90.00000000000000000, 95.00000000000000000, 3.000000000000000000 ) ) ;
#10427=AXIS2_PLACEMENT_3D ( 'NONE', #6568, #2915, #10314 ) ;
#10478=DIRECTION ( 'NONE',  ( 0.000000000000000000, 0.000000000000000000, -1.000000000000000000 ) ) ;
#10522=CYLINDRICAL_SURFACE ( 'NONE', #7595, 2.649999999999971934 ) ;
#10529=ORIENTED_EDGE ( 'NONE', *, *, #18498, .T. ) ;
#10536=FACE_OUTER_BOUND ( 'NONE', #10919, .T. ) ;
#10545=EDGE_CURVE ( 'NONE', #16945, #15162, #3654, .T. ) ;
#10557=CARTESIAN_POINT ( 'NONE',  ( -37.64999999999999147, 90.00000000000001421, 3.000000000000000000 ) ) ;
#10565=CARTESIAN_POINT ( 'NONE',  ( 110.0000000000000000, -74.99999999999998579, 0.000000000000000000 ) ) ;
#10567=CARTESIAN_POINT ( 'NONE',  ( 90.00000000000000000, 95.00000000000000000, 0.000000000000000000 ) ) ;
#10601=CARTESIAN_POINT ( 'NONE',  ( 93.00000000000000000, -149.9999999999996874, 129.9038105676659711 ) ) ;
#10613=ORIENTED_EDGE ( 'NONE', *, *, #2996, .T. ) ;
#10666=AXIS2_PLACEMENT_3D ( 'NONE', #13157, #15174, #11566 ) ;
#10707=ADVANCED_FACE ( 'NONE', ( #12054 ), #21403, .F. ) ;
#10724=ORIENTED_EDGE ( 'NONE', *, *, #4594, .T. ) ;
#10740=CARTESIAN_POINT ( 'NONE',  ( 93.00000000000000000, -74.99999999999998579, 129.9038105676659711 ) ) ;
#10752=DIRECTION ( 'NONE',  ( -0.000000000000000000, -0.000000000000000000, 1.000000000000000000 ) ) ;
#10758=ORIENTED_EDGE ( 'NONE', *, *, #23154, .T. ) ;
#10762=ORIENTED_EDGE ( 'NONE', *, *, #12244, .F. ) ;
#10790=AXIS2_PLACEMENT_3D ( 'NONE', #10254, #22797, #13562 ) ;
#10807=AXIS2_PLACEMENT_3D ( 'NONE', #1838, #18383, #12889 ) ;
#10815=AXIS2_PLACEMENT_3D ( 'NONE', #12449, #1276, #16268 ) ;
#10816=VERTEX_POINT ( 'NONE', #10095 ) ;
#10817=EDGE_CURVE ( 'NONE', #6073, #12669, #17436, .T. ) ;
#10818=DIRECTION ( 'NONE',  ( -0.000000000000000000, -0.000000000000000000, 1.000000000000000000 ) ) ;
#10837=VECTOR ( 'NONE', #6709, 1000.000000000000000 ) ;
#10855=ADVANCED_FACE ( 'NONE', ( #2656 ), #18823, .T. ) ;
#10886=DIRECTION ( 'NONE',  ( -0.000000000000000000, -0.000000000000000000, 1.000000000000000000 ) ) ;
#10898=LINE ( 'NONE', #16309, #1098 ) ;
#10903=ADVANCED_FACE ( 'NONE', ( #8222 ), #10056, .F. ) ;
#10906=DIRECTION ( 'NONE',  ( -1.000000000000000000, 7.709882115452476934E-17, 0.000000000000000000 ) ) ;
#10916=DIRECTION ( 'NONE',  ( 1.000000000000000000, 0.000000000000000000, 0.000000000000000000 ) ) ;
#10919=EDGE_LOOP ( 'NONE', ( #20212, #19671, #21060, #22883 ) ) ;
#10954=AXIS2_PLACEMENT_3D ( 'NONE', #10020, #23019, #13907 ) ;
#11023=CLOSED_SHELL ( 'NONE', ( #22089, #17418, #5593, #20988, #7260, #2378, #2773, #7518, #5435, #7473, #10855, #17566, #5203, #21279, #7522, #5290, #4376, #3245, #19834, #14448, #12255, #325, #10903, #138, #8081, #18891, #11383, #3248, #23308, #13174, #4731, #10707, #7482, #4848, #16249, #19964 ) ) ;
#11036=FACE_BOUND ( 'NONE', #8434, .T. ) ;
#11039=ORIENTED_EDGE ( 'NONE', *, *, #17933, .T. ) ;
#11074=EDGE_CURVE ( 'NONE', #13966, #16206, #9974, .T. ) ;
#11085=FACE_OUTER_BOUND ( 'NONE', #6930, .T. ) ;
#11128=ORIENTED_EDGE ( 'NONE', *, *, #4602, .F. ) ;
#11148=CARTESIAN_POINT ( 'NONE',  ( -110.0000000000000000, -94.99999999999997158, 0.000000000000000000 ) ) ;
#11171=CIRCLE ( 'NONE', #722, 2.649999999999971934 ) ;
#11193=AXIS2_PLACEMENT_3D ( 'NONE', #23357, #10478, #23233 ) ;
#11210=AXIS2_PLACEMENT_3D ( 'NONE', #9473, #14914, #3769 ) ;
#11229=EDGE_LOOP ( 'NONE', ( #9996, #4087 ) ) ;
#11233=COLOUR_RGB ( '',0.8941176470588234615, 0.8941176470588234615, 0.8941176470588234615 ) ;
#11255=EDGE_CURVE ( 'NONE', #7372, #13225, #17920, .T. ) ;
#11272=VERTEX_POINT ( 'NONE', #23223 ) ;
#11290=CARTESIAN_POINT ( 'NONE',  ( 93.00000000000000000, -149.9999999999996874, 129.9038105676659711 ) ) ;
#11291=CARTESIAN_POINT ( 'NONE',  ( -35.00000000000001421, 90.00000000000001421, 0.000000000000000000 ) ) ;
#11342=CARTESIAN_POINT ( 'NONE',  ( -110.0000000000000000, -94.99999999999997158, 3.000000000000000000 ) ) ;
#11383=ADVANCED_FACE ( 'NONE', ( #6030 ), #11639, .T. ) ;
#11399=EDGE_LOOP ( 'NONE', ( #15061, #21786 ) ) ;
#11438=LINE ( 'NONE', #2098, #9880 ) ;
#11458=VERTEX_POINT ( 'NONE', #6159 ) ;
#11471=ORIENTED_EDGE ( 'NONE', *, *, #23610, .F. ) ;
#11477=CARTESIAN_POINT ( 'NONE',  ( 37.64999999999996305, 90.00000000000000000, 0.000000000000000000 ) ) ;
#11491=VECTOR ( 'NONE', #16544, 1000.000000000000114 ) ;
#11507=CARTESIAN_POINT ( 'NONE',  ( -90.00000000000000000, 3.053113317719180486E-13, 129.9038105676659711 ) ) ;
#11513=DIRECTION ( 'NONE',  ( -0.000000000000000000, -0.000000000000000000, 1.000000000000000000 ) ) ;
#11516=CIRCLE ( 'NONE', #23037, 2.649999999999971934 ) ;
#11565=ORIENTED_EDGE ( 'NONE', *, *, #4107, .F. ) ;
#11566=DIRECTION ( 'NONE',  ( 0.000000000000000000, -0.000000000000000000, -1.000000000000000000 ) ) ;
#11576=VECTOR ( 'NONE', #4369, 1000.000000000000114 ) ;
#11639=PLANE ( 'NONE',  #13338 ) ;
#11657=DIRECTION ( 'NONE',  ( -1.000000000000000000, 0.000000000000000000, 0.000000000000000000 ) ) ;
#11669=DIRECTION ( 'NONE',  ( 1.000000000000000000, 0.000000000000000000, 0.000000000000000000 ) ) ;
#11675=ORIENTED_EDGE ( 'NONE', *, *, #12197, .T. ) ;
#11697=DIRECTION ( 'NONE',  ( 0.000000000000000000, 0.000000000000000000, -1.000000000000000000 ) ) ;
#11702=DIRECTION ( 'NONE',  ( 1.000000000000000000, 0.000000000000000000, 0.000000000000000000 ) ) ;
#11718=DIRECTION ( 'NONE',  ( 1.000000000000000000, 0.000000000000000000, 0.000000000000000000 ) ) ;
#11775=ORIENTED_EDGE ( 'NONE', *, *, #4602, .T. ) ;
#11777=CARTESIAN_POINT ( 'NONE',  ( 90.00000000000000000, -149.9999999999996874, 129.9038105676659711 ) ) ;
#11780=FACE_OUTER_BOUND ( 'NONE', #22422, .T. ) ;
#11797=CARTESIAN_POINT ( 'NONE',  ( -40.33333333333332860, -89.99999999999997158, 3.000000000000001332 ) ) ;
#11800=VECTOR ( 'NONE', #17238, 1000.000000000000000 ) ;
#11818=DIRECTION ( 'NONE',  ( 1.000000000000000000, 0.000000000000000000, 0.000000000000000000 ) ) ;
#11861=ORIENTED_EDGE ( 'NONE', *, *, #15487, .F. ) ;
#11872=LINE ( 'NONE', #19181, #16416 ) ;
#11885=MANIFOLD_SOLID_BREP ( 'M5 Clearance Hole1', #11023 ) ;
#11886=ORIENTED_EDGE ( 'NONE', *, *, #17470, .F. ) ;
#11916=VECTOR ( 'NONE', #13398, 1000.000000000000000 ) ;
#11939=CARTESIAN_POINT ( 'NONE',  ( 89.00000000000000000, -149.9999999999996874, 129.9038105676659711 ) ) ;
#11945=CARTESIAN_POINT ( 'NONE',  ( -90.00000000000000000, -94.99999999999998579, 0.000000000000000000 ) ) ;
#11946=VECTOR ( 'NONE', #2795, 1000.000000000000000 ) ;
#11949=CARTESIAN_POINT ( 'NONE',  ( 107.6499999999999773, 35.00000000000000000, 3.000000000000001332 ) ) ;
#11956=CARTESIAN_POINT ( 'NONE',  ( -35.00000000000001421, 90.00000000000001421, 3.000000000000000000 ) ) ;
#11958=VECTOR ( 'NONE', #15179, 1000.000000000000000 ) ;
#11965=VECTOR ( 'NONE', #16283, 1000.000000000000114 ) ;
#11975=VERTEX_POINT ( 'NONE', #20980 ) ;
#11989=AXIS2_PLACEMENT_3D ( 'NONE', #11507, #16914, #19069 ) ;
#12002=AXIS2_PLACEMENT_3D ( 'NONE', #3729, #22207, #5676 ) ;
#12013=CARTESIAN_POINT ( 'NONE',  ( 105.0000000000000000, -19.99999999999998934, 3.000000000000000000 ) ) ;
#12016=CARTESIAN_POINT ( 'NONE',  ( 89.00000000000000000, -94.99999999999998579, 0.000000000000000000 ) ) ;
#12054=FACE_OUTER_BOUND ( 'NONE', #10384, .T. ) ;
#12058=CARTESIAN_POINT ( 'NONE',  ( -107.6499999999999773, 30.00000000000001421, 3.000000000000000000 ) ) ;
#12098=CARTESIAN_POINT ( 'NONE',  ( -90.00000000000000000, -149.9999999999996874, 129.9038105676659711 ) ) ;
#12099=DIRECTION ( 'NONE',  ( 1.000000000000000000, 0.000000000000000000, 0.000000000000000000 ) ) ;
#12104=ORIENTED_EDGE ( 'NONE', *, *, #9418, .F. ) ;
#12175=ORIENTED_EDGE ( 'NONE', *, *, #13969, .T. ) ;
#12188=ORIENTED_EDGE ( 'NONE', *, *, #17138, .T. ) ;
#12197=EDGE_CURVE ( 'NONE', #301, #9146, #18635, .T. ) ;
#12212=DIRECTION ( 'NONE',  ( 1.000000000000000000, 0.000000000000000000, 0.000000000000000000 ) ) ;
#12223=PLANE ( 'NONE',  #935 ) ;
#12226=ORIENTED_EDGE ( 'NONE', *, *, #10545, .F. ) ;
#12244=EDGE_CURVE ( 'NONE', #6121, #15650, #2103, .T. ) ;
#12255=ADVANCED_FACE ( 'NONE', ( #20464 ), #13267, .F. ) ;
#12280=AXIS2_PLACEMENT_3D ( 'NONE', #16237, #14776, #23396 ) ;
#12291=EDGE_CURVE ( 'NONE', #16072, #16588, #19126, .T. ) ;
#12326=VERTEX_POINT ( 'NONE', #19002 ) ;
#12331=LINE ( 'NONE', #17041, #6717 ) ;
#12370=CARTESIAN_POINT ( 'NONE',  ( 89.00000000000000000, -74.99999999999998579, 0.000000000000000000 ) ) ;
#12398=ORIENTED_EDGE ( 'NONE', *, *, #23183, .T. ) ;
#12402=EDGE_CURVE ( 'NONE', #3284, #3058, #19848, .T. ) ;
#12410=LINE ( 'NONE', #10565, #14970 ) ;
#12412=LINE ( 'NONE', #10567, #20675 ) ;
#12416=AXIS2_PLACEMENT_3D ( 'NONE', #1408, #15924, #12212 ) ;
#12421=VERTEX_POINT ( 'NONE', #6696 ) ;
#12432=FACE_BOUND ( 'NONE', #13787, .T. ) ;
#12449=CARTESIAN_POINT ( 'NONE',  ( 0.000000000000000000, 0.000000000000000000, 0.000000000000000000 ) ) ;
#12464=EDGE_LOOP ( 'NONE', ( #13646, #4776 ) ) ;
#12474=CARTESIAN_POINT ( 'NONE',  ( -40.33333333333332860, -89.99999999999997158, 0.000000000000000000 ) ) ;
#12510=ORIENTED_EDGE ( 'NONE', *, *, #17385, .F. ) ;
#12520=AXIS2_PLACEMENT_3D ( 'NONE', #21671, #5821, #1381 ) ;
#12556=CARTESIAN_POINT ( 'NONE',  ( -90.00000000000000000, -74.99999999999998579, 0.000000000000000000 ) ) ;
#12560=CARTESIAN_POINT ( 'NONE',  ( -90.00000000000000000, 3.053113317719180486E-13, 3.000000000000002665 ) ) ;
#12570=LINE ( 'NONE', #16384, #11965 ) ;
#12571=DIRECTION ( 'NONE',  ( 0.000000000000000000, 0.000000000000000000, 1.000000000000000000 ) ) ;
#12584=CARTESIAN_POINT ( 'NONE',  ( -102.3500000000000227, 30.00000000000001421, 3.000000000000001332 ) ) ;
#12590=CARTESIAN_POINT ( 'NONE',  ( 105.0000000000000000, 35.00000000000000000, 3.000000000000000000 ) ) ;
#12614=CARTESIAN_POINT ( 'NONE',  ( -93.00000000000000000, 76.26794919243116055, 2.999999999999988898 ) ) ;
#12640=CARTESIAN_POINT ( 'NONE',  ( 105.0000000000000000, 35.00000000000000000, 3.000000000000000000 ) ) ;
#12669=VERTEX_POINT ( 'NONE', #248 ) ;
#12718=ORIENTED_EDGE ( 'NONE', *, *, #7978, .T. ) ;
#12763=CARTESIAN_POINT ( 'NONE',  ( 107.6499999999999631, 35.00000000000000000, 3.000000000000000000 ) ) ;
#12765=EDGE_CURVE ( 'NONE', #16072, #9980, #12331, .T. ) ;
#12801=VECTOR ( 'NONE', #19344, 1000.000000000000000 ) ;
#12851=ORIENTED_EDGE ( 'NONE', *, *, #16367, .F. ) ;
#12853=CARTESIAN_POINT ( 'NONE',  ( -35.00000000000001421, 90.00000000000001421, 3.000000000000001332 ) ) ;
#12880=AXIS2_PLACEMENT_3D ( 'NONE', #17129, #6263, #15213 ) ;
#12889=DIRECTION ( 'NONE',  ( 0.000000000000000000, 0.000000000000000000, -1.000000000000000000 ) ) ;
#12895=CARTESIAN_POINT ( 'NONE',  ( 105.0000000000000000, -19.99999999999998934, 0.000000000000000000 ) ) ;
#12908=ORIENTED_EDGE ( 'NONE', *, *, #3731, .T. ) ;
#12911=CARTESIAN_POINT ( 'NONE',  ( -110.0000000000000142, 95.00000000000001421, 3.000000000000000000 ) ) ;
#12924=MECHANICAL_DESIGN_GEOMETRIC_PRESENTATION_REPRESENTATION('',(#20193),#15227);
#12974=LINE ( 'NONE', #5682, #17708 ) ;
#13018=AXIS2_PLACEMENT_3D ( 'NONE', #7504, #7991, #22359 ) ;
#13045=DIRECTION ( 'NONE',  ( 0.000000000000000000, 1.000000000000000000, 0.000000000000000000 ) ) ;
#13057=DIRECTION ( 'NONE',  ( 1.000000000000000000, 0.000000000000000000, 0.000000000000000000 ) ) ;
#13107=CARTESIAN_POINT ( 'NONE',  ( 32.35000000000001563, 90.00000000000000000, 0.000000000000000000 ) ) ;
#13111=STYLED_ITEM ( 'NONE', ( #13334 ), #8186 ) ;
#13118=VECTOR ( 'NONE', #19819, 1000.000000000000000 ) ;
#13157=CARTESIAN_POINT ( 'NONE',  ( 110.0000000000000000, -74.99999999999998579, 3.000000000000000000 ) ) ;
#13174=ADVANCED_FACE ( 'NONE', ( #1146 ), #8525, .F. ) ;
#13202=EDGE_CURVE ( 'NONE', #2178, #16805, #15611, .T. ) ;
#13215=ORIENTED_EDGE ( 'NONE', *, *, #2996, .F. ) ;
#13223=EDGE_LOOP ( 'NONE', ( #4077, #14105, #15838, #12175 ) ) ;
#13225=VERTEX_POINT ( 'NONE', #18167 ) ;
#13257=DIRECTION ( 'NONE',  ( -0.000000000000000000, -0.000000000000000000, 1.000000000000000000 ) ) ;
#13267=PLANE ( 'NONE',  #2487 ) ;
#13269=FACE_OUTER_BOUND ( 'NONE', #8056, .T. ) ;
#13288=VECTOR ( 'NONE', #23593, 1000.000000000000000 ) ;
#13303=CARTESIAN_POINT ( 'NONE',  ( -105.0000000000000000, -29.99999999999998579, 3.000000000000000000 ) ) ;
#13334=PRESENTATION_STYLE_ASSIGNMENT (( #5927 ) ) ;
#13338=AXIS2_PLACEMENT_3D ( 'NONE', #16674, #2036, #20753 ) ;
#13367=LINE ( 'NONE', #5719, #22674 ) ;
#13376=CARTESIAN_POINT ( 'NONE',  ( 26.98333333333332007, -89.99999999999998579, 3.000000000000001332 ) ) ;
#13385=AXIS2_PLACEMENT_3D ( 'NONE', #11797, #13257, #22744 ) ;
#13398=DIRECTION ( 'NONE',  ( -1.000000000000000000, 7.709882115452476934E-17, 0.000000000000000000 ) ) ;
#13435=CIRCLE ( 'NONE', #12280, 2.649999999999985700 ) ;
#13479=ORIENTED_EDGE ( 'NONE', *, *, #7745, .F. ) ;
#13494=CARTESIAN_POINT ( 'NONE',  ( -102.3500000000000369, 30.00000000000001421, 3.000000000000000000 ) ) ;
#13504=CARTESIAN_POINT ( 'NONE',  ( 90.00000000000000000, 3.000000000000293987, 129.9038105676659711 ) ) ;
#13545=EDGE_CURVE ( 'NONE', #20480, #10816, #13836, .T. ) ;
#13550=VERTEX_POINT ( 'NONE', #528 ) ;
#13562=DIRECTION ( 'NONE',  ( 1.000000000000000000, 0.000000000000000000, 0.000000000000000000 ) ) ;
#13601=CARTESIAN_POINT ( 'NONE',  ( -40.33333333333332860, -89.99999999999997158, 3.000000000000000000 ) ) ;
#13603=EDGE_CURVE ( 'NONE', #12326, #14560, #19098, .T. ) ;
#13617=CARTESIAN_POINT ( 'NONE',  ( 90.00000000000000000, 76.26794919243113213, 3.000000000000002665 ) ) ;
#13646=ORIENTED_EDGE ( 'NONE', *, *, #9316, .F. ) ;
#13688=ORIENTED_EDGE ( 'NONE', *, *, #13545, .F. ) ;
#13699=( NAMED_UNIT ( * ) PLANE_ANGLE_UNIT ( ) SI_UNIT ( $, .RADIAN. ) );
#13717=EDGE_CURVE ( 'NONE', #11975, #15717, #5332, .T. ) ;
#13746=ORIENTED_EDGE ( 'NONE', *, *, #22567, .F. ) ;
#13787=EDGE_LOOP ( 'NONE', ( #21028, #11471 ) ) ;
#13792=DIRECTION ( 'NONE',  ( -7.709882115452476934E-17, -1.000000000000000000, 0.000000000000000000 ) ) ;
#13812=CIRCLE ( 'NONE', #272, 2.649999999999971934 ) ;
#13836=LINE ( 'NONE', #4621, #6899 ) ;
#13870=LINE ( 'NONE', #21313, #17318 ) ;
#13907=DIRECTION ( 'NONE',  ( -1.000000000000000000, 0.000000000000000000, 0.000000000000000000 ) ) ;
#13914=CIRCLE ( 'NONE', #23112, 2.649999999999985700 ) ;
#13924=ORIENTED_EDGE ( 'NONE', *, *, #23003, .F. ) ;
#13959=FACE_OUTER_BOUND ( 'NONE', #14292, .T. ) ;
#13966=VERTEX_POINT ( 'NONE', #14647 ) ;
#13969=EDGE_CURVE ( 'NONE', #17494, #1219, #12974, .T. ) ;
#13980=ORIENTED_EDGE ( 'NONE', *, *, #16662, .T. ) ;
#13999=DIRECTION ( 'NONE',  ( -0.000000000000000000, -0.000000000000000000, 1.000000000000000000 ) ) ;
#14096=CIRCLE ( 'NONE', #3625, 2.649999999999985700 ) ;
#14105=ORIENTED_EDGE ( 'NONE', *, *, #12291, .F. ) ;
#14106=CIRCLE ( 'NONE', #3637, 2.649999999999989253 ) ;
#14139=CIRCLE ( 'NONE', #22190, 2.649999999999971934 ) ;
#14148=CARTESIAN_POINT ( 'NONE',  ( 90.00000000000000000, -74.99999999999998579, 0.000000000000000000 ) ) ;
#14170=DIRECTION ( 'NONE',  ( -0.000000000000000000, -0.000000000000000000, 1.000000000000000000 ) ) ;
#14181=AXIS2_PLACEMENT_3D ( 'NONE', #12474, #23535, #3120 ) ;
#14214=FACE_BOUND ( 'NONE', #5976, .T. ) ;
#14218=CARTESIAN_POINT ( 'NONE',  ( -110.0000000000000142, 95.00000000000001421, 0.000000000000000000 ) ) ;
#14260=CIRCLE ( 'NONE', #6143, 2.649999999999985700 ) ;
#14261=EDGE_CURVE ( 'NONE', #6335, #6867, #10009, .T. ) ;
#14279=LINE ( 'NONE', #2771, #23157 ) ;
#14282=VECTOR ( 'NONE', #8848, 1000.000000000000000 ) ;
#14292=EDGE_LOOP ( 'NONE', ( #4329, #714, #23538, #4381 ) ) ;
#14310=CARTESIAN_POINT ( 'NONE',  ( 110.0000000000000000, -74.99999999999998579, 3.000000000000000000 ) ) ;
#14312=VECTOR ( 'NONE', #5030, 1000.000000000000000 ) ;
#14342=FACE_BOUND ( 'NONE', #5500, .T. ) ;
#14376=CARTESIAN_POINT ( 'NONE',  ( 90.00000000000000000, -149.9999999999996874, 129.9038105676659711 ) ) ;
#14395=EDGE_CURVE ( 'NONE', #10091, #10816, #4316, .T. ) ;
#14407=DIRECTION ( 'NONE',  ( 0.000000000000000000, -0.8660254037844398178, -0.4999999999999980016 ) ) ;
#14409=FACE_OUTER_BOUND ( 'NONE', #4030, .T. ) ;
#14448=ADVANCED_FACE ( 'NONE', ( #6721, #2954, #3319, #8913, #17829, #16142, #23506, #21330, #1397 ), #16375, .T. ) ;
#14459=ORIENTED_EDGE ( 'NONE', *, *, #901, .F. ) ;
#14461=FACE_OUTER_BOUND ( 'NONE', #2372, .T. ) ;
#14501=EDGE_CURVE ( 'NONE', #17898, #7277, #18065, .T. ) ;
#14503=AXIS2_PLACEMENT_3D ( 'NONE', #23008, #19750, #21332 ) ;
#14551=DIRECTION ( 'NONE',  ( 0.000000000000000000, -1.000000000000000000, 0.000000000000000000 ) ) ;
#14560=VERTEX_POINT ( 'NONE', #15929 ) ;
#14620=DIRECTION ( 'NONE',  ( 0.000000000000000000, 1.000000000000000000, 0.000000000000000000 ) ) ;
#14639=CARTESIAN_POINT ( 'NONE',  ( -105.0000000000000142, 30.00000000000001421, 3.000000000000000000 ) ) ;
#14647=CARTESIAN_POINT ( 'NONE',  ( 89.00000000000000000, -74.99999999999998579, 3.000000000000000000 ) ) ;
#14662=AXIS2_PLACEMENT_3D ( 'NONE', #13601, #16758, #13057 ) ;
#14676=CIRCLE ( 'NONE', #2697, 2.649999999999985700 ) ;
#14694=VECTOR ( 'NONE', #1433, 1000.000000000000000 ) ;
#14728=ORIENTED_EDGE ( 'NONE', *, *, #19191, .T. ) ;
#14776=DIRECTION ( 'NONE',  ( -0.000000000000000000, -0.000000000000000000, 1.000000000000000000 ) ) ;
#14781=EDGE_CURVE ( 'NONE', #2736, #21146, #5636, .T. ) ;
#14851=VECTOR ( 'NONE', #2585, 1000.000000000000114 ) ;
#14868=VECTOR ( 'NONE', #4704, 1000.000000000000000 ) ;
#14869=EDGE_CURVE ( 'NONE', #11458, #6121, #16998, .T. ) ;
#14873=CARTESIAN_POINT ( 'NONE',  ( 93.00000000000000000, -149.9999999999996874, 129.9038105676659711 ) ) ;
#14880=ORIENTED_EDGE ( 'NONE', *, *, #17627, .F. ) ;
#14914=DIRECTION ( 'NONE',  ( 0.000000000000000000, 0.000000000000000000, 1.000000000000000000 ) ) ;
#14932=PLANE ( 'NONE',  #10666 ) ;
#14970=VECTOR ( 'NONE', #21761, 1000.000000000000000 ) ;
#14973=CARTESIAN_POINT ( 'NONE',  ( -90.00000000000000000, -74.99999999999998579, 3.000000000000000000 ) ) ;
#15059=VECTOR ( 'NONE', #13045, 1000.000000000000000 ) ;
#15061=ORIENTED_EDGE ( 'NONE', *, *, #6196, .F. ) ;
#15086=EDGE_CURVE ( 'NONE', #10091, #5513, #4536, .T. ) ;
#15087=VERTEX_POINT ( 'NONE', #11949 ) ;
#15156=ORIENTED_EDGE ( 'NONE', *, *, #10372, .T. ) ;
#15162=VERTEX_POINT ( 'NONE', #19490 ) ;
#15174=DIRECTION ( 'NONE',  ( 0.000000000000000000, -1.000000000000000000, 0.000000000000000000 ) ) ;
#15175=FACE_OUTER_BOUND ( 'NONE', #6243, .T. ) ;
#15176=ORIENTED_EDGE ( 'NONE', *, *, #13545, .T. ) ;
#15179=DIRECTION ( 'NONE',  ( -0.000000000000000000, -0.000000000000000000, 1.000000000000000000 ) ) ;
#15199=CARTESIAN_POINT ( 'NONE',  ( 107.6499999999999631, -19.99999999999998934, 3.000000000000000000 ) ) ;
#15213=DIRECTION ( 'NONE',  ( 1.000000000000000000, 0.000000000000000000, 0.000000000000000000 ) ) ;
#15218=VERTEX_POINT ( 'NONE', #5374 ) ;
#15227=( GEOMETRIC_REPRESENTATION_CONTEXT ( 3 ) GLOBAL_UNCERTAINTY_ASSIGNED_CONTEXT ( ( #17255 ) ) GLOBAL_UNIT_ASSIGNED_CONTEXT ( ( #7946, #18790, #4192 ) ) REPRESENTATION_CONTEXT ( 'NONE', 'WORKASPACE' ) );
#15233=VERTEX_POINT ( 'NONE', #16472 ) ;
#15256=VERTEX_POINT ( 'NONE', #17077 ) ;
#15275=EDGE_LOOP ( 'NONE', ( #836, #10277, #10758, #4751 ) ) ;
#15286=ORIENTED_EDGE ( 'NONE', *, *, #10817, .F. ) ;
#15295=DIRECTION ( 'NONE',  ( -0.000000000000000000, -1.000000000000000000, 0.000000000000000000 ) ) ;
#15296=CYLINDRICAL_SURFACE ( 'NONE', #977, 2.649999999999971934 ) ;
#15300=DIRECTION ( 'NONE',  ( -0.000000000000000000, -0.000000000000000000, 1.000000000000000000 ) ) ;
#15332=CARTESIAN_POINT ( 'NONE',  ( -90.00000000000000000, -149.9999999999996874, 129.9038105676659711 ) ) ;
#15396=DIRECTION ( 'NONE',  ( -0.000000000000000000, -0.000000000000000000, 1.000000000000000000 ) ) ;
#15436=CARTESIAN_POINT ( 'NONE',  ( 90.00000000000000000, 2.914335439641035919E-13, 129.9038105676659711 ) ) ;
#15460=EDGE_CURVE ( 'NONE', #1219, #6867, #21294, .T. ) ;
#15487=EDGE_CURVE ( 'NONE', #13550, #17898, #8369, .T. ) ;
#15514=ORIENTED_EDGE ( 'NONE', *, *, #5849, .F. ) ;
#15527=EDGE_CURVE ( 'NONE', #16945, #3284, #12410, .T. ) ;
#15556=AXIS2_PLACEMENT_3D ( 'NONE', #13303, #8080, #4069 ) ;
#15590=ORIENTED_EDGE ( 'NONE', *, *, #16734, .F. ) ;
#15611=CIRCLE ( 'NONE', #2856, 2.649999999999989253 ) ;
#15650=VERTEX_POINT ( 'NONE', #508 ) ;
#15661=VERTEX_POINT ( 'NONE', #13107 ) ;
#15677=EDGE_CURVE ( 'NONE', #4839, #20854, #11516, .T. ) ;
#15695=DIRECTION ( 'NONE',  ( -0.000000000000000000, 1.000000000000000000, 0.000000000000000000 ) ) ;
#15717=VERTEX_POINT ( 'NONE', #6291 ) ;
#15735=CARTESIAN_POINT ( 'NONE',  ( -107.6499999999999773, 30.00000000000001421, 0.000000000000000000 ) ) ;
#15765=LINE ( 'NONE', #21422, #9182 ) ;
#15818=VECTOR ( 'NONE', #15695, 1000.000000000000000 ) ;
#15838=ORIENTED_EDGE ( 'NONE', *, *, #18903, .F. ) ;
#15872=ORIENTED_EDGE ( 'NONE', *, *, #17738, .F. ) ;
#15888=CARTESIAN_POINT ( 'NONE',  ( 24.33333333333333215, -89.99999999999998579, 0.000000000000000000 ) ) ;
#15891=ORIENTED_EDGE ( 'NONE', *, *, #6638, .T. ) ;
#15894=ORIENTED_EDGE ( 'NONE', *, *, #23154, .F. ) ;
#15924=DIRECTION ( 'NONE',  ( -0.000000000000000000, -0.000000000000000000, 1.000000000000000000 ) ) ;
#15929=CARTESIAN_POINT ( 'NONE',  ( -107.6499999999999773, -29.99999999999998579, 3.000000000000001332 ) ) ;
#15940=EDGE_LOOP ( 'NONE', ( #8998, #17031 ) ) ;
#15956=( LENGTH_UNIT ( ) NAMED_UNIT ( * ) SI_UNIT ( .MILLI., .METRE. ) );
#15961=ORIENTED_EDGE ( 'NONE', *, *, #994, .F. ) ;
#15989=CARTESIAN_POINT ( 'NONE',  ( -93.00000000000000000, -79.73205080756885366, 3.000000000000002665 ) ) ;
#16020=CARTESIAN_POINT ( 'NONE',  ( -93.00000000000000000, 3.053113317719180486E-13, 3.000000000000002665 ) ) ;
#16021=CARTESIAN_POINT ( 'NONE',  ( 89.00000000000000000, -76.73205080756885366, 3.000000000000000000 ) ) ;
#16052=DIRECTION ( 'NONE',  ( 1.000000000000000000, -7.709882115452476934E-17, 0.000000000000000000 ) ) ;
#16072=VERTEX_POINT ( 'NONE', #20717 ) ;
#16085=ORIENTED_EDGE ( 'NONE', *, *, #14395, .F. ) ;
#16128=DIRECTION ( 'NONE',  ( 0.000000000000000000, 0.000000000000000000, -1.000000000000000000 ) ) ;
#16142=FACE_BOUND ( 'NONE', #11399, .T. ) ;
#16145=LINE ( 'NONE', #12560, #18830 ) ;
#16164=AXIS2_PLACEMENT_3D ( 'NONE', #3916, #11697, #9497 ) ;
#16206=VERTEX_POINT ( 'NONE', #16021 ) ;
#16211=ORIENTED_EDGE ( 'NONE', *, *, #10545, .T. ) ;
#16219=CARTESIAN_POINT ( 'NONE',  ( 89.00000000000000000, -79.73205080756883945, 2.999999999999988898 ) ) ;
#16223=EDGE_LOOP ( 'NONE', ( #2233, #7076, #21105, #15286 ) ) ;
#16237=CARTESIAN_POINT ( 'NONE',  ( 105.0000000000000000, 35.00000000000000000, 3.000000000000001332 ) ) ;
#16249=ADVANCED_FACE ( 'NONE', ( #6602 ), #21084, .F. ) ;
#16251=DIRECTION ( 'NONE',  ( -1.000000000000000000, 0.000000000000000000, 0.000000000000000000 ) ) ;
#16268=DIRECTION ( 'NONE',  ( -1.000000000000000000, 0.000000000000000000, -0.000000000000000000 ) ) ;
#16269=ORIENTED_EDGE ( 'NONE', *, *, #18498, .F. ) ;
#16271=DIRECTION ( 'NONE',  ( -1.000000000000000000, -0.000000000000000000, 0.000000000000000000 ) ) ;
#16283=DIRECTION ( 'NONE',  ( -0.000000000000000000, 0.4999999999999979461, -0.8660254037844397068 ) ) ;
#16309=CARTESIAN_POINT ( 'NONE',  ( -42.98333333333330586, -89.99999999999997158, 3.000000000000000000 ) ) ;
#16316=AXIS2_PLACEMENT_3D ( 'NONE', #12013, #6521, #19422 ) ;
#16326=DIRECTION ( 'NONE',  ( -0.000000000000000000, -0.000000000000000000, 1.000000000000000000 ) ) ;
#16340=LINE ( 'NONE', #12763, #21442 ) ;
#16367=EDGE_CURVE ( 'NONE', #11975, #1617, #19863, .T. ) ;
#16375=PLANE ( 'NONE',  #10815 ) ;
#16384=CARTESIAN_POINT ( 'NONE',  ( 89.00000000000000000, -152.9999999999996874, 129.9038105676659711 ) ) ;
#16388=VERTEX_POINT ( 'NONE', #69 ) ;
#16405=EDGE_CURVE ( 'NONE', #4707, #23406, #20271, .T. ) ;
#16416=VECTOR ( 'NONE', #17398, 1000.000000000000000 ) ;
#16417=SHAPE_DEFINITION_REPRESENTATION ( #1879, #21947 ) ;
#16432=FACE_OUTER_BOUND ( 'NONE', #5704, .T. ) ;
#16435=ORIENTED_EDGE ( 'NONE', *, *, #3197, .F. ) ;
#16472=CARTESIAN_POINT ( 'NONE',  ( -37.68333333333335844, -89.99999999999997158, 0.000000000000000000 ) ) ;
#16518=VECTOR ( 'NONE', #14551, 1000.000000000000000 ) ;
#16525=ORIENTED_EDGE ( 'NONE', *, *, #5930, .T. ) ;
#16544=DIRECTION ( 'NONE',  ( -0.000000000000000000, 0.4999999999999979461, -0.8660254037844397068 ) ) ;
#16549=AXIS2_PLACEMENT_3D ( 'NONE', #9740, #15300, #9618 ) ;
#16579=EDGE_CURVE ( 'NONE', #13966, #7277, #17798, .T. ) ;
#16588=VERTEX_POINT ( 'NONE', #15989 ) ;
#16658=CARTESIAN_POINT ( 'NONE',  ( -32.35000000000002984, 90.00000000000001421, 3.000000000000001332 ) ) ;
#16662=EDGE_CURVE ( 'NONE', #15218, #15087, #16340, .T. ) ;
#16674=CARTESIAN_POINT ( 'NONE',  ( -90.00000000000000000, -74.99999999999998579, 3.000000000000000000 ) ) ;
#16704=VECTOR ( 'NONE', #6461, 1000.000000000000000 ) ;
#16721=ORIENTED_EDGE ( 'NONE', *, *, #16734, .T. ) ;
#16730=LINE ( 'NONE', #661, #5247 ) ;
#16734=EDGE_CURVE ( 'NONE', #15162, #9146, #12412, .T. ) ;
#16758=DIRECTION ( 'NONE',  ( -0.000000000000000000, -0.000000000000000000, 1.000000000000000000 ) ) ;
#16769=VECTOR ( 'NONE', #1272, 1000.000000000000000 ) ;
#16796=FACE_BOUND ( 'NONE', #21536, .T. ) ;
#16797=EDGE_CURVE ( 'NONE', #12326, #6747, #5655, .T. ) ;
#16804=DIRECTION ( 'NONE',  ( 0.000000000000000000, 0.000000000000000000, -1.000000000000000000 ) ) ;
#16805=VERTEX_POINT ( 'NONE', #9701 ) ;
#16808=CIRCLE ( 'NONE', #14503, 2.649999999999985700 ) ;
#16821=EDGE_CURVE ( 'NONE', #20854, #4839, #9527, .T. ) ;
#16839=DIRECTION ( 'NONE',  ( 1.000000000000000000, 0.000000000000000000, 0.000000000000000000 ) ) ;
#16844=CARTESIAN_POINT ( 'NONE',  ( 34.99999999999999289, 90.00000000000000000, 0.000000000000000000 ) ) ;
#16846=CARTESIAN_POINT ( 'NONE',  ( 110.0000000000000000, -74.99999999999998579, 3.000000000000000000 ) ) ;
#16890=VECTOR ( 'NONE', #17358, 1000.000000000000000 ) ;
#16914=DIRECTION ( 'NONE',  ( 1.000000000000000000, 0.000000000000000000, 0.000000000000000000 ) ) ;
#16932=( GEOMETRIC_REPRESENTATION_CONTEXT ( 3 ) GLOBAL_UNCERTAINTY_ASSIGNED_CONTEXT ( ( #18789 ) ) GLOBAL_UNIT_ASSIGNED_CONTEXT ( ( #15956, #8467, #23297 ) ) REPRESENTATION_CONTEXT ( 'NONE', 'WORKASPACE' ) );
#16945=VERTEX_POINT ( 'NONE', #1217 ) ;
#16952=CIRCLE ( 'NONE', #21597, 2.649999999999985700 ) ;
#16956=CIRCLE ( 'NONE', #9646, 2.649999999999971934 ) ;
#16986=LINE ( 'NONE', #7794, #11958 ) ;
#16998=LINE ( 'NONE', #9389, #22734 ) ;
#17031=ORIENTED_EDGE ( 'NONE', *, *, #16405, .F. ) ;
#17041=CARTESIAN_POINT ( 'NONE',  ( -90.00000000000000000, -152.9999999999996874, 129.9038105676659711 ) ) ;
#17063=FACE_OUTER_BOUND ( 'NONE', #13223, .T. ) ;
#17076=DIRECTION ( 'NONE',  ( 1.000000000000000000, 0.000000000000000000, 0.000000000000000000 ) ) ;
#17077=CARTESIAN_POINT ( 'NONE',  ( 107.6499999999999773, -19.99999999999998934, 3.000000000000001332 ) ) ;
#17095=EDGE_CURVE ( 'NONE', #6335, #17494, #3599, .T. ) ;
#17129=CARTESIAN_POINT ( 'NONE',  ( 24.33333333333333215, -89.99999999999998579, 3.000000000000000000 ) ) ;
#17138=EDGE_CURVE ( 'NONE', #11458, #13550, #18461, .T. ) ;
#17145=VECTOR ( 'NONE', #194, 1000.000000000000000 ) ;
#17173=CARTESIAN_POINT ( 'NONE',  ( -40.33333333333332860, -89.99999999999997158, 0.000000000000000000 ) ) ;
#17203=AXIS2_PLACEMENT_3D ( 'NONE', #21034, #9581, #8243 ) ;
#17204=PLANE ( 'NONE',  #1442 ) ;
#17209=DIRECTION ( 'NONE',  ( 0.000000000000000000, -1.000000000000000000, 0.000000000000000000 ) ) ;
#17222=DIRECTION ( 'NONE',  ( 1.000000000000000000, 0.000000000000000000, 0.000000000000000000 ) ) ;
#17238=DIRECTION ( 'NONE',  ( -0.000000000000000000, -0.000000000000000000, 1.000000000000000000 ) ) ;
#17254=PLANE ( 'NONE',  #2794 ) ;
#17255=UNCERTAINTY_MEASURE_WITH_UNIT (LENGTH_MEASURE( 1.000000000000000082E-05 ), #7946, 'distance_accuracy_value', 'NONE');
#17262=CARTESIAN_POINT ( 'NONE',  ( -110.0000000000000142, 95.00000000000001421, 3.000000000000000000 ) ) ;
#17305=DIRECTION ( 'NONE',  ( 0.000000000000000000, 0.000000000000000000, 1.000000000000000000 ) ) ;
#17318=VECTOR ( 'NONE', #19256, 1000.000000000000000 ) ;
#17348=DIRECTION ( 'NONE',  ( 1.000000000000000000, 0.000000000000000000, 0.000000000000000000 ) ) ;
#17349=CARTESIAN_POINT ( 'NONE',  ( 102.3500000000000085, -19.99999999999998934, 3.000000000000001332 ) ) ;
#17358=DIRECTION ( 'NONE',  ( -0.000000000000000000, -1.000000000000000000, 0.000000000000000000 ) ) ;
#17385=EDGE_CURVE ( 'NONE', #4839, #7372, #10148, .T. ) ;
#17398=DIRECTION ( 'NONE',  ( -1.000000000000000000, 7.709882115452476934E-17, 0.000000000000000000 ) ) ;
#17401=VERTEX_POINT ( 'NONE', #12584 ) ;
#17408=ORIENTED_EDGE ( 'NONE', *, *, #22252, .T. ) ;
#17418=ADVANCED_FACE ( 'NONE', ( #5417 ), #10522, .F. ) ;
#17436=LINE ( 'NONE', #17797, #23113 ) ;
#17450=CARTESIAN_POINT ( 'NONE',  ( -32.35000000000004405, 90.00000000000001421, 0.000000000000000000 ) ) ;
#17470=EDGE_CURVE ( 'NONE', #15233, #19530, #655, .T. ) ;
#17480=VECTOR ( 'NONE', #5629, 1000.000000000000000 ) ;
#17481=DIRECTION ( 'NONE',  ( -1.000000000000000000, 0.000000000000000000, 0.000000000000000000 ) ) ;
#17494=VERTEX_POINT ( 'NONE', #23750 ) ;
#17566=ADVANCED_FACE ( 'NONE', ( #20935 ), #17204, .F. ) ;
#17610=AXIS2_PLACEMENT_3D ( 'NONE', #22579, #11513, #4478 ) ;
#17627=EDGE_CURVE ( 'NONE', #20433, #20414, #17640, .T. ) ;
#17640=CIRCLE ( 'NONE', #7229, 2.649999999999971934 ) ;
#17648=EDGE_LOOP ( 'NONE', ( #22688, #5341, #10613, #9153 ) ) ;
#17673=DIRECTION ( 'NONE',  ( -0.000000000000000000, -0.000000000000000000, 1.000000000000000000 ) ) ;
#17680=DIRECTION ( 'NONE',  ( -0.000000000000000000, -0.000000000000000000, 1.000000000000000000 ) ) ;
#17708=VECTOR ( 'NONE', #21990, 1000.000000000000114 ) ;
#17738=EDGE_CURVE ( 'NONE', #20433, #7876, #996, .T. ) ;
#17797=CARTESIAN_POINT ( 'NONE',  ( 37.64999999999996305, 90.00000000000000000, 3.000000000000000000 ) ) ;
#17798=LINE ( 'NONE', #19458, #8345 ) ;
#17802=DIRECTION ( 'NONE',  ( -0.000000000000000000, -0.000000000000000000, 1.000000000000000000 ) ) ;
#17821=ORIENTED_EDGE ( 'NONE', *, *, #9056, .F. ) ;
#17829=FACE_BOUND ( 'NONE', #12464, .T. ) ;
#17885=PRODUCT ( 'discharge spout', 'discharge spout', '', ( #18794 ) ) ;
#17898=VERTEX_POINT ( 'NONE', #1955 ) ;
#17906=AXIS2_PLACEMENT_3D ( 'NONE', #1680, #14620, #7015 ) ;
#17920=CIRCLE ( 'NONE', #7497, 2.649999999999985700 ) ;
#17929=CARTESIAN_POINT ( 'NONE',  ( 105.0000000000000000, -19.99999999999998934, 3.000000000000001332 ) ) ;
#17933=EDGE_CURVE ( 'NONE', #15087, #12421, #13435, .T. ) ;
#17947=DIRECTION ( 'NONE',  ( 1.000000000000000000, 0.000000000000000000, 0.000000000000000000 ) ) ;
#17988=CARTESIAN_POINT ( 'NONE',  ( -110.0000000000000000, 75.00000000000001421, 3.000000000000000000 ) ) ;
#18007=CARTESIAN_POINT ( 'NONE',  ( 93.00000000000000000, -149.9999999999996874, 129.9038105676659711 ) ) ;
#18010=DIRECTION ( 'NONE',  ( 0.000000000000000000, -0.4999999999999979461, 0.8660254037844397068 ) ) ;
#18038=EDGE_LOOP ( 'NONE', ( #7342, #1410, #9975, #4088 ) ) ;
#18065=LINE ( 'NONE', #12556, #1143 ) ;
#18079=CARTESIAN_POINT ( 'NONE',  ( 26.98333333333330231, -89.99999999999998579, 0.000000000000000000 ) ) ;
#18081=AXIS2_PLACEMENT_3D ( 'NONE', #8916, #16271, #23616 ) ;
#18102=DIRECTION ( 'NONE',  ( 1.000000000000000000, 0.000000000000000000, 0.000000000000000000 ) ) ;
#18105=CYLINDRICAL_SURFACE ( 'NONE', #22559, 2.649999999999971934 ) ;
#18108=ORIENTED_EDGE ( 'NONE', *, *, #16579, .F. ) ;
#18166=CARTESIAN_POINT ( 'NONE',  ( 89.00000000000000000, -149.9999999999996874, 129.9038105676659711 ) ) ;
#18167=CARTESIAN_POINT ( 'NONE',  ( -37.65000000000000568, 90.00000000000001421, 3.000000000000001332 ) ) ;
#18178=CARTESIAN_POINT ( 'NONE',  ( 110.0000000000000000, -74.99999999999998579, 3.000000000000000000 ) ) ;
#18188=DIRECTION ( 'NONE',  ( -0.000000000000000000, 1.000000000000000000, 0.000000000000000000 ) ) ;
#18196=CYLINDRICAL_SURFACE ( 'NONE', #12416, 2.649999999999971934 ) ;
#18197=CARTESIAN_POINT ( 'NONE',  ( 90.00000000000000000, 75.00000000000000000, 0.000000000000000000 ) ) ;
#18207=ORIENTED_EDGE ( 'NONE', *, *, #12402, .T. ) ;
#18358=DIRECTION ( 'NONE',  ( -0.000000000000000000, -0.000000000000000000, -1.000000000000000000 ) ) ;
#18383=DIRECTION ( 'NONE',  ( 1.000000000000000000, 0.000000000000000000, 0.000000000000000000 ) ) ;
#18404=CIRCLE ( 'NONE', #8803, 2.649999999999971934 ) ;
#18461=LINE ( 'NONE', #2276, #11491 ) ;
#18471=CIRCLE ( 'NONE', #11193, 2.649999999999971934 ) ;
#18498=EDGE_CURVE ( 'NONE', #1617, #15162, #19384, .T. ) ;
#18555=EDGE_CURVE ( 'NONE', #21242, #12669, #16808, .T. ) ;
#18599=DIRECTION ( 'NONE',  ( -1.000000000000000000, 0.000000000000000000, 0.000000000000000000 ) ) ;
#18635=LINE ( 'NONE', #12911, #17145 ) ;
#18664=VECTOR ( 'NONE', #16839, 1000.000000000000000 ) ;
#18727=ORIENTED_EDGE ( 'NONE', *, *, #14501, .T. ) ;
#18756=DIRECTION ( 'NONE',  ( 1.000000000000000000, 0.000000000000000000, 0.000000000000000000 ) ) ;
#18773=ORIENTED_EDGE ( 'NONE', *, *, #5930, .F. ) ;
#18774=EDGE_LOOP ( 'NONE', ( #3021, #8777, #18773, #11675 ) ) ;
#18789=UNCERTAINTY_MEASURE_WITH_UNIT (LENGTH_MEASURE( 1.000000000000000082E-05 ), #15956, 'distance_accuracy_value', 'NONE');
#18790=( NAMED_UNIT ( * ) PLANE_ANGLE_UNIT ( ) SI_UNIT ( $, .RADIAN. ) );
#18794=PRODUCT_CONTEXT ( 'NONE', #22932, 'mechanical' ) ;
#18796=DIRECTION ( 'NONE',  ( -0.000000000000000000, -0.000000000000000000, -1.000000000000000000 ) ) ;
#18797=DIRECTION ( 'NONE',  ( 0.000000000000000000, 0.4999999999999980016, -0.8660254037844397068 ) ) ;
#18804=CIRCLE ( 'NONE', #19194, 2.649999999999985700 ) ;
#18814=ORIENTED_EDGE ( 'NONE', *, *, #14869, .T. ) ;
#18815=ORIENTED_EDGE ( 'NONE', *, *, #21226, .T. ) ;
#18823=PLANE ( 'NONE',  #11989 ) ;
#18830=VECTOR ( 'NONE', #18188, 1000.000000000000000 ) ;
#18835=ORIENTED_EDGE ( 'NONE', *, *, #17470, .T. ) ;
#18850=EDGE_CURVE ( 'NONE', #20480, #16588, #16730, .T. ) ;
#18891=ADVANCED_FACE ( 'NONE', ( #6223 ), #14932, .T. ) ;
#18903=EDGE_CURVE ( 'NONE', #17494, #16072, #11438, .T. ) ;
#18928=FACE_OUTER_BOUND ( 'NONE', #2416, .T. ) ;
#18931=ORIENTED_EDGE ( 'NONE', *, *, #9436, .T. ) ;
#18932=EDGE_CURVE ( 'NONE', #15661, #6073, #14139, .T. ) ;
#18944=EDGE_LOOP ( 'NONE', ( #16721, #151, #11128, #10529 ) ) ;
#18977=DIRECTION ( 'NONE',  ( 0.000000000000000000, -1.000000000000000000, 0.000000000000000000 ) ) ;
#18990=EDGE_CURVE ( 'NONE', #17401, #7876, #16952, .T. ) ;
#19002=CARTESIAN_POINT ( 'NONE',  ( -107.6499999999999631, -29.99999999999998579, 0.000000000000000000 ) ) ;
#19007=DIRECTION ( 'NONE',  ( -0.000000000000000000, -0.000000000000000000, 1.000000000000000000 ) ) ;
#19042=ORIENTED_EDGE ( 'NONE', *, *, #20545, .F. ) ;
#19069=DIRECTION ( 'NONE',  ( 0.000000000000000000, 0.000000000000000000, -1.000000000000000000 ) ) ;
#19093=PLANE ( 'NONE',  #7556 ) ;
#19098=LINE ( 'NONE', #19336, #11946 ) ;
#19118=ORIENTED_EDGE ( 'NONE', *, *, #11074, .F. ) ;
#19126=LINE ( 'NONE', #22765, #14851 ) ;
#19132=CARTESIAN_POINT ( 'NONE',  ( -105.0000000000000000, -29.99999999999998579, 3.000000000000000000 ) ) ;
#19137=LINE ( 'NONE', #5869, #16890 ) ;
#19149=EDGE_CURVE ( 'NONE', #6073, #15661, #22352, .T. ) ;
#19163=FACE_OUTER_BOUND ( 'NONE', #17648, .T. ) ;
#19181=CARTESIAN_POINT ( 'NONE',  ( 90.00000000000000000, 95.00000000000000000, 3.000000000000000000 ) ) ;
#19191=EDGE_CURVE ( 'NONE', #22443, #2736, #20401, .T. ) ;
#19194=AXIS2_PLACEMENT_3D ( 'NONE', #9862, #9621, #17348 ) ;
#19201=ORIENTED_EDGE ( 'NONE', *, *, #15487, .T. ) ;
#19207=VECTOR ( 'NONE', #18796, 1000.000000000000000 ) ;
#19216=EDGE_LOOP ( 'NONE', ( #23325, #15176, #12398, #5745, #18108, #9693, #7453, #6652 ) ) ;
#19256=DIRECTION ( 'NONE',  ( 1.000000000000000000, 0.000000000000000000, 0.000000000000000000 ) ) ;
#19260=CARTESIAN_POINT ( 'NONE',  ( 21.68333333333335844, -89.99999999999998579, 3.000000000000000000 ) ) ;
#19285=PRODUCT_DEFINITION_FORMATION_WITH_SPECIFIED_SOURCE ( 'ANY', '', #17885, .NOT_KNOWN. ) ;
#19314=CYLINDRICAL_SURFACE ( 'NONE', #16316, 2.649999999999971934 ) ;
#19336=CARTESIAN_POINT ( 'NONE',  ( -107.6499999999999631, -29.99999999999998579, 3.000000000000000000 ) ) ;
#19344=DIRECTION ( 'NONE',  ( 1.000000000000000000, -7.709882115452475701E-17, 0.000000000000000000 ) ) ;
#19384=LINE ( 'NONE', #19633, #10245 ) ;
#19422=DIRECTION ( 'NONE',  ( 1.000000000000000000, 0.000000000000000000, 0.000000000000000000 ) ) ;
#19456=DIRECTION ( 'NONE',  ( -1.000000000000000000, 0.000000000000000000, -0.000000000000000000 ) ) ;
#19458=CARTESIAN_POINT ( 'NONE',  ( 89.00000000000000000, -74.99999999999998579, 3.000000000000000000 ) ) ;
#19490=CARTESIAN_POINT ( 'NONE',  ( 110.0000000000000000, 95.00000000000000000, 0.000000000000000000 ) ) ;
#19530=VERTEX_POINT ( 'NONE', #9893 ) ;
#19633=CARTESIAN_POINT ( 'NONE',  ( 110.0000000000000000, 95.00000000000000000, 3.000000000000000000 ) ) ;
#19634=LINE ( 'NONE', #1171, #6131 ) ;
#19639=DIRECTION ( 'NONE',  ( -0.000000000000000000, -0.000000000000000000, 1.000000000000000000 ) ) ;
#19671=ORIENTED_EDGE ( 'NONE', *, *, #1340, .T. ) ;
#19694=DIRECTION ( 'NONE',  ( -0.000000000000000000, 0.8660254037844398178, 0.4999999999999980016 ) ) ;
#19736=LINE ( 'NONE', #19260, #10341 ) ;
#19747=VERTEX_POINT ( 'NONE', #3204 ) ;
#19750=DIRECTION ( 'NONE',  ( -0.000000000000000000, -0.000000000000000000, 1.000000000000000000 ) ) ;
#19769=ORIENTED_EDGE ( 'NONE', *, *, #4035, .T. ) ;
#19819=DIRECTION ( 'NONE',  ( -1.000000000000000000, 0.000000000000000000, 0.000000000000000000 ) ) ;
#19834=ADVANCED_FACE ( 'NONE', ( #11085 ), #22511, .F. ) ;
#19848=LINE ( 'NONE', #19959, #13288 ) ;
#19856=CARTESIAN_POINT ( 'NONE',  ( -105.0000000000000142, 30.00000000000001421, 0.000000000000000000 ) ) ;
#19863=LINE ( 'NONE', #18178, #21066 ) ;
#19902=DIRECTION ( 'NONE',  ( -0.000000000000000000, -0.000000000000000000, 1.000000000000000000 ) ) ;
#19914=EDGE_CURVE ( 'NONE', #23021, #20709, #8084, .T. ) ;
#19921=ORIENTED_EDGE ( 'NONE', *, *, #8485, .F. ) ;
#19956=ORIENTED_EDGE ( 'NONE', *, *, #18903, .T. ) ;
#19959=CARTESIAN_POINT ( 'NONE',  ( 93.00000000000000000, -74.99999999999998579, 0.000000000000000000 ) ) ;
#19964=ADVANCED_FACE ( 'NONE', ( #13269 ), #20577, .F. ) ;
#19966=EDGE_CURVE ( 'NONE', #15661, #21242, #16986, .T. ) ;
#20056=DIRECTION ( 'NONE',  ( 1.000000000000000000, 0.000000000000000000, 0.000000000000000000 ) ) ;
#20182=DIRECTION ( 'NONE',  ( 0.000000000000000000, 0.000000000000000000, -1.000000000000000000 ) ) ;
#20193=STYLED_ITEM('',(#23934),#11885);
#20197=PLANE ( 'NONE',  #10807 ) ;
#20202=DIRECTION ( 'NONE',  ( -1.000000000000000000, 0.000000000000000000, 0.000000000000000000 ) ) ;
#20207=DIRECTION ( 'NONE',  ( 1.000000000000000000, 0.000000000000000000, 0.000000000000000000 ) ) ;
#20212=ORIENTED_EDGE ( 'NONE', *, *, #9316, .T. ) ;
#20222=EDGE_CURVE ( 'NONE', #7277, #8336, #4263, .T. ) ;
#20270=ORIENTED_EDGE ( 'NONE', *, *, #14501, .F. ) ;
#20271=CIRCLE ( 'NONE', #13385, 2.649999999999985700 ) ;
#20332=ORIENTED_EDGE ( 'NONE', *, *, #9042, .F. ) ;
#20401=LINE ( 'NONE', #14873, #23521 ) ;
#20402=VECTOR ( 'NONE', #11718, 1000.000000000000000 ) ;
#20414=VERTEX_POINT ( 'NONE', #10184 ) ;
#20433=VERTEX_POINT ( 'NONE', #15735 ) ;
#20464=FACE_OUTER_BOUND ( 'NONE', #3028, .T. ) ;
#20466=EDGE_LOOP ( 'NONE', ( #13479, #5164, #8401, #12188 ) ) ;
#20480=VERTEX_POINT ( 'NONE', #16219 ) ;
#20484=ORIENTED_EDGE ( 'NONE', *, *, #13202, .T. ) ;
#20523=CARTESIAN_POINT ( 'NONE',  ( 93.00000000000000000, 76.26794919243113213, 2.999999999999975131 ) ) ;
#20545=EDGE_CURVE ( 'NONE', #14560, #442, #8417, .T. ) ;
#20556=ORIENTED_EDGE ( 'NONE', *, *, #7978, .F. ) ;
#20572=DIRECTION ( 'NONE',  ( -1.000000000000000000, 0.000000000000000000, 0.000000000000000000 ) ) ;
#20575=DIRECTION ( 'NONE',  ( 0.000000000000000000, 0.000000000000000000, 1.000000000000000000 ) ) ;
#20577=CYLINDRICAL_SURFACE ( 'NONE', #16549, 2.649999999999971934 ) ;
#20649=ORIENTED_EDGE ( 'NONE', *, *, #18932, .T. ) ;
#20675=VECTOR ( 'NONE', #1358, 1000.000000000000000 ) ;
#20685=DIRECTION ( 'NONE',  ( 0.000000000000000000, 0.4999999999999979461, -0.8660254037844397068 ) ) ;
#20709=VERTEX_POINT ( 'NONE', #18079 ) ;
#20717=CARTESIAN_POINT ( 'NONE',  ( -93.00000000000000000, -152.9999999999996874, 129.9038105676659711 ) ) ;
#20753=DIRECTION ( 'NONE',  ( 0.000000000000000000, -0.000000000000000000, 1.000000000000000000 ) ) ;
#20779=CARTESIAN_POINT ( 'NONE',  ( -35.00000000000001421, 90.00000000000001421, 0.000000000000000000 ) ) ;
#20785=DIRECTION ( 'NONE',  ( -1.000000000000000000, 0.000000000000000000, 0.000000000000000000 ) ) ;
#20786=CIRCLE ( 'NONE', #10790, 2.649999999999985700 ) ;
#20799=CARTESIAN_POINT ( 'NONE',  ( 89.00000000000000000, -74.99999999999998579, 0.000000000000000000 ) ) ;
#20832=ORIENTED_EDGE ( 'NONE', *, *, #9436, .F. ) ;
#20843=CYLINDRICAL_SURFACE ( 'NONE', #5344, 2.649999999999971934 ) ;
#20851=DIRECTION ( 'NONE',  ( 0.000000000000000000, -1.000000000000000000, 0.000000000000000000 ) ) ;
#20854=VERTEX_POINT ( 'NONE', #9270 ) ;
#20935=FACE_OUTER_BOUND ( 'NONE', #565, .T. ) ;
#20954=DIRECTION ( 'NONE',  ( -0.000000000000000000, -0.000000000000000000, 1.000000000000000000 ) ) ;
#20980=CARTESIAN_POINT ( 'NONE',  ( 110.0000000000000000, -74.99999999999998579, 3.000000000000000000 ) ) ;
#20988=ADVANCED_FACE ( 'NONE', ( #557 ), #20843, .F. ) ;
#21017=ORIENTED_EDGE ( 'NONE', *, *, #15460, .T. ) ;
#21020=ORIENTED_EDGE ( 'NONE', *, *, #8285, .F. ) ;
#21028=ORIENTED_EDGE ( 'NONE', *, *, #21226, .F. ) ;
#21034=CARTESIAN_POINT ( 'NONE',  ( -93.00000000000000000, 3.053113317719180486E-13, 129.9038105676659711 ) ) ;
#21049=DIRECTION ( 'NONE',  ( 0.000000000000000000, -1.000000000000000000, 0.000000000000000000 ) ) ;
#21060=ORIENTED_EDGE ( 'NONE', *, *, #23610, .T. ) ;
#21063=CARTESIAN_POINT ( 'NONE',  ( -105.0000000000000142, 30.00000000000001421, 3.000000000000001332 ) ) ;
#21066=VECTOR ( 'NONE', #5377, 1000.000000000000000 ) ;
#21074=DIRECTION ( 'NONE',  ( -0.000000000000000000, -0.000000000000000000, 1.000000000000000000 ) ) ;
#21084=CYLINDRICAL_SURFACE ( 'NONE', #6484, 2.649999999999971934 ) ;
#21105=ORIENTED_EDGE ( 'NONE', *, *, #18555, .T. ) ;
#21110=ORIENTED_EDGE ( 'NONE', *, *, #8229, .F. ) ;
#21146=VERTEX_POINT ( 'NONE', #1262 ) ;
#21152=ORIENTED_EDGE ( 'NONE', *, *, #18850, .T. ) ;
#21200=CARTESIAN_POINT ( 'NONE',  ( -40.33333333333332860, -89.99999999999997158, 3.000000000000000000 ) ) ;
#21218=EDGE_CURVE ( 'NONE', #6121, #5073, #13870, .T. ) ;
#21222=DIRECTION ( 'NONE',  ( -0.000000000000000000, 0.4999999999999979461, -0.8660254037844397068 ) ) ;
#21226=EDGE_CURVE ( 'NONE', #15256, #6626, #14260, .T. ) ;
#21242=VERTEX_POINT ( 'NONE', #5021 ) ;
#21279=ADVANCED_FACE ( 'NONE', ( #9239 ), #20197, .T. ) ;
#21294=LINE ( 'NONE', #13617, #12801 ) ;
#21313=CARTESIAN_POINT ( 'NONE',  ( -90.00000000000000000, -149.9999999999996874, 129.9038105676659711 ) ) ;
#21330=FACE_BOUND ( 'NONE', #5581, .T. ) ;
#21332=DIRECTION ( 'NONE',  ( 1.000000000000000000, 0.000000000000000000, 0.000000000000000000 ) ) ;
#21399=CARTESIAN_POINT ( 'NONE',  ( -90.00000000000000000, 75.00000000000001421, 0.000000000000000000 ) ) ;
#21403=CYLINDRICAL_SURFACE ( 'NONE', #10427, 2.649999999999971934 ) ;
#21422=CARTESIAN_POINT ( 'NONE',  ( -90.00000000000000000, -76.73205080756885366, 3.000000000000002665 ) ) ;
#21442=VECTOR ( 'NONE', #10818, 1000.000000000000000 ) ;
#21473=ORIENTED_EDGE ( 'NONE', *, *, #22276, .F. ) ;
#21536=EDGE_LOOP ( 'NONE', ( #4739, #15961 ) ) ;
#21551=AXIS2_PLACEMENT_3D ( 'NONE', #12640, #17802, #6928 ) ;
#21594=EDGE_CURVE ( 'NONE', #11975, #16945, #8969, .T. ) ;
#21597=AXIS2_PLACEMENT_3D ( 'NONE', #21063, #17673, #2819 ) ;
#21611=EDGE_LOOP ( 'NONE', ( #13688, #21152, #15156, #21017, #23007, #7561, #8344, #11775, #16525, #4572 ) ) ;
#21623=DIRECTION ( 'NONE',  ( 0.000000000000000000, -1.000000000000000000, 0.000000000000000000 ) ) ;
#21639=CARTESIAN_POINT ( 'NONE',  ( -90.00000000000000000, -152.9999999999996874, 129.9038105676659711 ) ) ;
#21644=ORIENTED_EDGE ( 'NONE', *, *, #13969, .F. ) ;
#21657=ORIENTED_EDGE ( 'NONE', *, *, #23003, .T. ) ;
#21658=DIRECTION ( 'NONE',  ( -1.000000000000000000, 0.000000000000000000, 0.000000000000000000 ) ) ;
#21667=CARTESIAN_POINT ( 'NONE',  ( 93.00000000000000000, -149.9999999999996874, 129.9038105676659711 ) ) ;
#21671=CARTESIAN_POINT ( 'NONE',  ( 0.000000000000000000, 0.000000000000000000, 3.000000000000000000 ) ) ;
#21713=DIRECTION ( 'NONE',  ( 1.000000000000000000, 0.000000000000000000, 0.000000000000000000 ) ) ;
#21722=CARTESIAN_POINT ( 'NONE',  ( -42.98333333333332007, -89.99999999999997158, 3.000000000000001332 ) ) ;
#21726=ORIENTED_EDGE ( 'NONE', *, *, #843, .T. ) ;
#21749=DIRECTION ( 'NONE',  ( -0.000000000000000000, -0.000000000000000000, 1.000000000000000000 ) ) ;
#21758=AXIS2_PLACEMENT_3D ( 'NONE', #21200, #19007, #2474 ) ;
#21761=DIRECTION ( 'NONE',  ( -1.000000000000000000, 0.000000000000000000, 0.000000000000000000 ) ) ;
#21786=ORIENTED_EDGE ( 'NONE', *, *, #7623, .F. ) ;
#21800=PLANE ( 'NONE',  #7726 ) ;
#21811=LINE ( 'NONE', #10740, #6289 ) ;
#21825=CARTESIAN_POINT ( 'NONE',  ( 24.33333333333333215, -89.99999999999998579, 3.000000000000001332 ) ) ;
#21853=CYLINDRICAL_SURFACE ( 'NONE', #1545, 2.649999999999971934 ) ;
#21935=VECTOR ( 'NONE', #18358, 1000.000000000000000 ) ;
#21947=SHAPE_REPRESENTATION ( 'discharge spout', ( #11210 ), #22754 ) ;
#21984=ORIENTED_EDGE ( 'NONE', *, *, #3731, .F. ) ;
#21990=DIRECTION ( 'NONE',  ( -0.000000000000000000, 0.4999999999999979461, -0.8660254037844397068 ) ) ;
#22057=CARTESIAN_POINT ( 'NONE',  ( -105.0000000000000142, 30.00000000000001421, 0.000000000000000000 ) ) ;
#22082=DIRECTION ( 'NONE',  ( 1.000000000000000000, 0.000000000000000000, 0.000000000000000000 ) ) ;
#22089=ADVANCED_FACE ( 'NONE', ( #1404 ), #8662, .F. ) ;
#22190=AXIS2_PLACEMENT_3D ( 'NONE', #16844, #302, #20572 ) ;
#22207=DIRECTION ( 'NONE',  ( 0.000000000000000000, 0.000000000000000000, -1.000000000000000000 ) ) ;
#22252=EDGE_CURVE ( 'NONE', #5073, #16206, #6339, .T. ) ;
#22265=DIRECTION ( 'NONE',  ( -1.000000000000000000, 0.000000000000000000, 0.000000000000000000 ) ) ;
#22276=EDGE_CURVE ( 'NONE', #12669, #21242, #18804, .T. ) ;
#22313=DIRECTION ( 'NONE',  ( -0.000000000000000000, -0.000000000000000000, 1.000000000000000000 ) ) ;
#22352=CIRCLE ( 'NONE', #12002, 2.649999999999971934 ) ;
#22359=DIRECTION ( 'NONE',  ( -1.000000000000000000, 0.000000000000000000, 0.000000000000000000 ) ) ;
#22366=ORIENTED_EDGE ( 'NONE', *, *, #14261, .T. ) ;
#22396=CARTESIAN_POINT ( 'NONE',  ( -90.00000000000000000, -149.9999999999996874, 129.9038105676659711 ) ) ;
#22397=ORIENTED_EDGE ( 'NONE', *, *, #3086, .T. ) ;
#22422=EDGE_LOOP ( 'NONE', ( #9717, #4547, #9544, #22397 ) ) ;
#22436=EDGE_CURVE ( 'NONE', #16206, #15650, #15765, .T. ) ;
#22443=VERTEX_POINT ( 'NONE', #21667 ) ;
#22501=ORIENTED_EDGE ( 'NONE', *, *, #21594, .T. ) ;
#22511=PLANE ( 'NONE',  #16164 ) ;
#22545=PLANE ( 'NONE',  #3171 ) ;
#22559=AXIS2_PLACEMENT_3D ( 'NONE', #12590, #19902, #1559 ) ;
#22567=EDGE_CURVE ( 'NONE', #5073, #9980, #7517, .T. ) ;
#22579=CARTESIAN_POINT ( 'NONE',  ( -105.0000000000000000, -29.99999999999998579, 3.000000000000001332 ) ) ;
#22586=DIRECTION ( 'NONE',  ( 0.000000000000000000, 0.000000000000000000, -1.000000000000000000 ) ) ;
#22651=ORIENTED_EDGE ( 'NONE', *, *, #17627, .T. ) ;
#22674=VECTOR ( 'NONE', #9361, 1000.000000000000000 ) ;
#22688=ORIENTED_EDGE ( 'NONE', *, *, #13603, .F. ) ;
#22708=EDGE_CURVE ( 'NONE', #23406, #4707, #1476, .T. ) ;
#22721=FACE_OUTER_BOUND ( 'NONE', #34, .T. ) ;
#22734=VECTOR ( 'NONE', #20851, 1000.000000000000000 ) ;
#22744=DIRECTION ( 'NONE',  ( 1.000000000000000000, 0.000000000000000000, 0.000000000000000000 ) ) ;
#22754=( GEOMETRIC_REPRESENTATION_CONTEXT ( 3 ) GLOBAL_UNCERTAINTY_ASSIGNED_CONTEXT ( ( #9946 ) ) GLOBAL_UNIT_ASSIGNED_CONTEXT ( ( #2539, #13699, #9696 ) ) REPRESENTATION_CONTEXT ( 'NONE', 'WORKASPACE' ) );
#22765=CARTESIAN_POINT ( 'NONE',  ( -93.00000000000000000, -152.9999999999996874, 129.9038105676659711 ) ) ;
#22771=DIRECTION ( 'NONE',  ( -0.000000000000000000, -0.000000000000000000, 1.000000000000000000 ) ) ;
#22797=DIRECTION ( 'NONE',  ( -0.000000000000000000, -0.000000000000000000, 1.000000000000000000 ) ) ;
#22798=CYLINDRICAL_SURFACE ( 'NONE', #12880, 2.649999999999971934 ) ;
#22826=EDGE_LOOP ( 'NONE', ( #5059, #2215, #18931, #20484 ) ) ;
#22838=EDGE_CURVE ( 'NONE', #19530, #4707, #10898, .T. ) ;
#22857=ORIENTED_EDGE ( 'NONE', *, *, #994, .T. ) ;
#22881=CARTESIAN_POINT ( 'NONE',  ( -110.0000000000000000, -94.99999999999997158, 3.000000000000000000 ) ) ;
#22883=ORIENTED_EDGE ( 'NONE', *, *, #1724, .F. ) ;
#22896=ORIENTED_EDGE ( 'NONE', *, *, #22276, .T. ) ;
#22932=APPLICATION_CONTEXT ( 'automotive_design' ) ;
#22941=CARTESIAN_POINT ( 'NONE',  ( -35.00000000000001421, 90.00000000000001421, 3.000000000000001332 ) ) ;
#22970=DIRECTION ( 'NONE',  ( -0.000000000000000000, -0.000000000000000000, 1.000000000000000000 ) ) ;
#23003=EDGE_CURVE ( 'NONE', #11272, #17898, #4068, .T. ) ;
#23007=ORIENTED_EDGE ( 'NONE', *, *, #5849, .T. ) ;
#23008=CARTESIAN_POINT ( 'NONE',  ( 34.99999999999999289, 90.00000000000000000, 3.000000000000001332 ) ) ;
#23019=DIRECTION ( 'NONE',  ( 0.000000000000000000, 0.000000000000000000, -1.000000000000000000 ) ) ;
#23021=VERTEX_POINT ( 'NONE', #7581 ) ;
#23037=AXIS2_PLACEMENT_3D ( 'NONE', #11291, #16804, #18599 ) ;
#23112=AXIS2_PLACEMENT_3D ( 'NONE', #2477, #21074, #17222 ) ;
#23113=VECTOR ( 'NONE', #878, 1000.000000000000000 ) ;
#23154=EDGE_CURVE ( 'NONE', #12421, #15087, #20786, .T. ) ;
#23157=VECTOR ( 'NONE', #21623, 1000.000000000000000 ) ;
#23183=EDGE_CURVE ( 'NONE', #10816, #8336, #8201, .T. ) ;
#23223=CARTESIAN_POINT ( 'NONE',  ( -90.00000000000000000, -74.99999999999998579, 3.000000000000002665 ) ) ;
#23233=DIRECTION ( 'NONE',  ( -1.000000000000000000, 0.000000000000000000, 0.000000000000000000 ) ) ;
#23260=FACE_OUTER_BOUND ( 'NONE', #22826, .T. ) ;
#23278=CARTESIAN_POINT ( 'NONE',  ( -35.00000000000001421, 90.00000000000001421, 3.000000000000000000 ) ) ;
#23297=( NAMED_UNIT ( * ) SI_UNIT ( $, .STERADIAN. ) SOLID_ANGLE_UNIT ( ) );
#23298=ORIENTED_EDGE ( 'NONE', *, *, #22436, .F. ) ;
#23299=EDGE_CURVE ( 'NONE', #9980, #20480, #12570, .T. ) ;
#23308=ADVANCED_FACE ( 'NONE', ( #23260 ), #18196, .F. ) ;
#23325=ORIENTED_EDGE ( 'NONE', *, *, #23299, .T. ) ;
#23357=CARTESIAN_POINT ( 'NONE',  ( -105.0000000000000000, -29.99999999999998579, 0.000000000000000000 ) ) ;
#23378=DIRECTION ( 'NONE',  ( -0.000000000000000000, 0.4999999999999979461, -0.8660254037844397068 ) ) ;
#23396=DIRECTION ( 'NONE',  ( 1.000000000000000000, 0.000000000000000000, 0.000000000000000000 ) ) ;
#23397=EDGE_LOOP ( 'NONE', ( #9288, #15891, #22857, #12510 ) ) ;
#23406=VERTEX_POINT ( 'NONE', #3563 ) ;
#23425=ORIENTED_EDGE ( 'NONE', *, *, #2389, .T. ) ;
#23446=ORIENTED_EDGE ( 'NONE', *, *, #7623, .T. ) ;
#23506=FACE_BOUND ( 'NONE', #7911, .T. ) ;
#23521=VECTOR ( 'NONE', #3865, 1000.000000000000000 ) ;
#23535=DIRECTION ( 'NONE',  ( 0.000000000000000000, 0.000000000000000000, -1.000000000000000000 ) ) ;
#23538=ORIENTED_EDGE ( 'NONE', *, *, #12765, .F. ) ;
#23541=FACE_OUTER_BOUND ( 'NONE', #1649, .T. ) ;
#23557=PLANE ( 'NONE',  #17906 ) ;
#23593=DIRECTION ( 'NONE',  ( -1.000000000000000000, 0.000000000000000000, 0.000000000000000000 ) ) ;
#23610=EDGE_CURVE ( 'NONE', #6626, #15256, #13914, .T. ) ;
#23616=DIRECTION ( 'NONE',  ( 0.000000000000000000, 0.000000000000000000, 1.000000000000000000 ) ) ;
#23657=LINE ( 'NONE', #1677, #8769 ) ;
#23679=ORIENTED_EDGE ( 'NONE', *, *, #15527, .T. ) ;
#23693=ORIENTED_EDGE ( 'NONE', *, *, #7707, .T. ) ;
#23698=ORIENTED_EDGE ( 'NONE', *, *, #7707, .F. ) ;
#23750=CARTESIAN_POINT ( 'NONE',  ( -93.00000000000000000, 3.000000000000308198, 129.9038105676659711 ) ) ;
#23772=EDGE_CURVE ( 'NONE', #6747, #12326, #18471, .T. ) ;
#23928=COLOUR_RGB('Off White',0.89,0.88,0.83);
#23929=FILL_AREA_STYLE_COLOUR('',#23928);
#23930=FILL_AREA_STYLE('',(#23929));
#23931=SURFACE_STYLE_FILL_AREA(#23930);
#23932=SURFACE_SIDE_STYLE('',(#23931));
#23933=SURFACE_STYLE_USAGE(.BOTH.,#23932);
#23934=PRESENTATION_STYLE_ASSIGNMENT((#23933));
ENDSEC;
END-ISO-10303-21;
